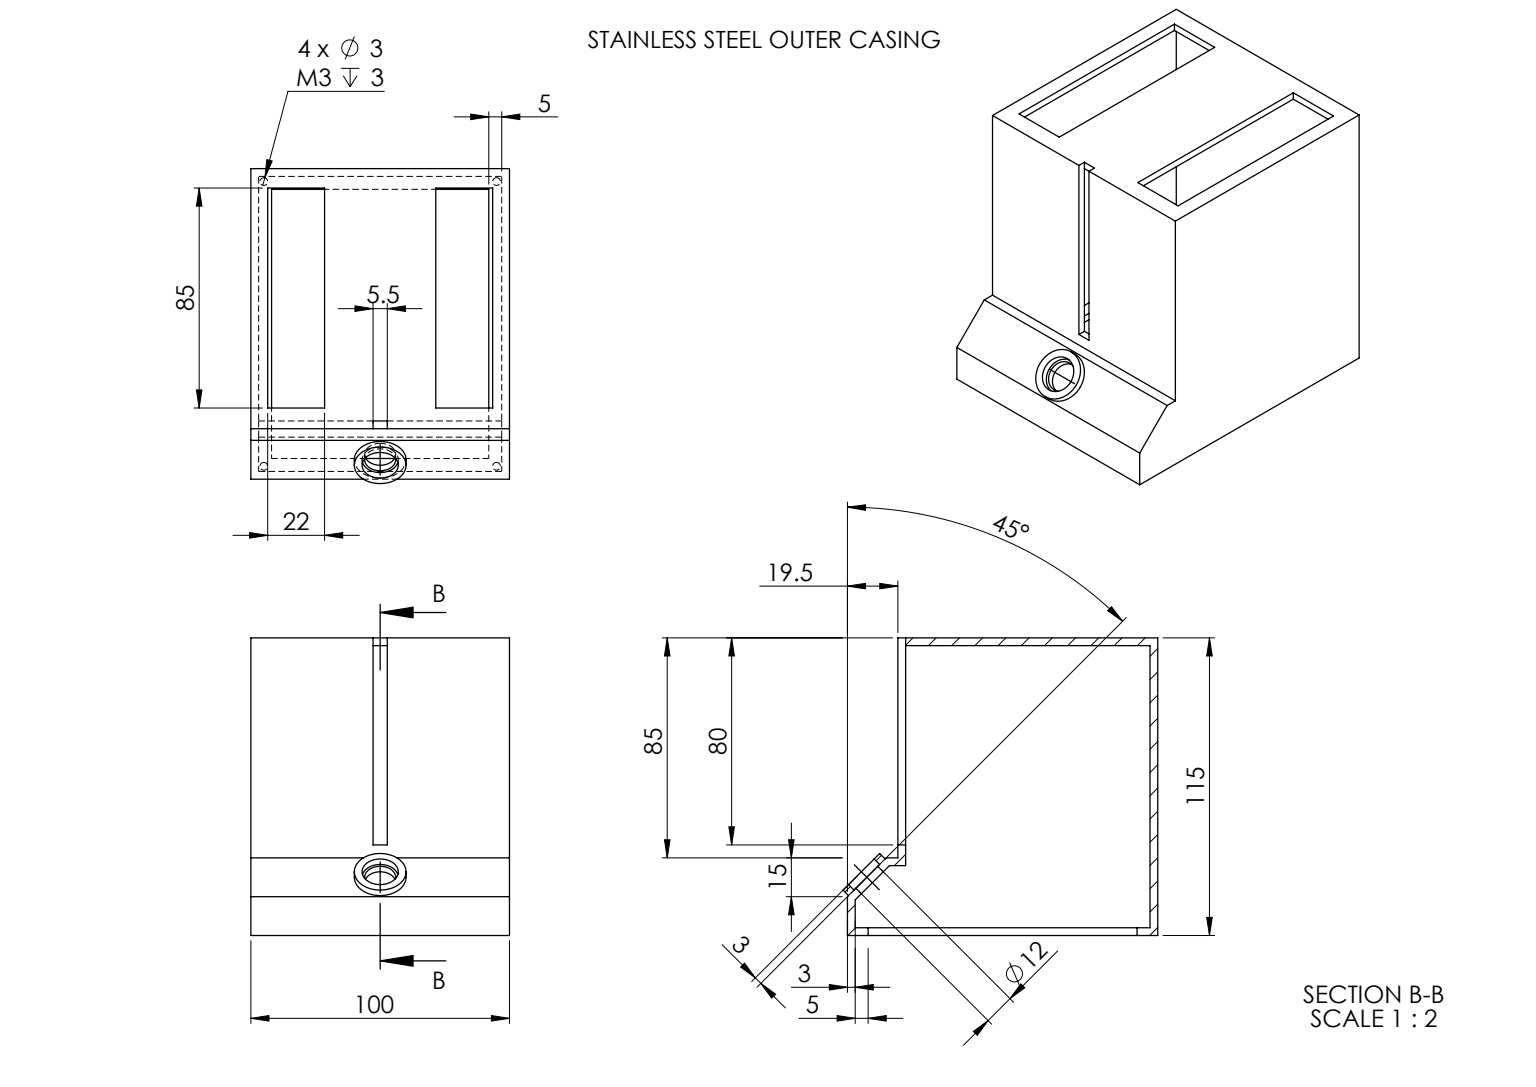
ISO-10303-21;
HEADER;
FILE_DESCRIPTION (('STEP AP214'),
    '1' );
FILE_NAME ('Stainless Steel Outer Casing.step',
    '2026-10-08T14:41:38',
    ( '' ),
    ( '' ),
    'SwSTEP 2.0',
    'SolidWorks 2026',
    '' );
FILE_SCHEMA (( 'AUTOMOTIVE_DESIGN' ));
ENDSEC;

DATA;
#7=VECTOR ( 'NONE', #15495, 1000.000000000000000 ) ;
#21=EDGE_CURVE ( 'NONE', #10175, #2143, #13600, .T. ) ;
#32=VECTOR ( 'NONE', #13036, 1000.000000000000114 ) ;
#63=VECTOR ( 'NONE', #9225, 1000.000000000000114 ) ;
#94=FACE_OUTER_BOUND ( 'NONE', #15883, .T. ) ;
#99=CARTESIAN_POINT ( 'NONE',  ( 44.99999999999997158, 6.000000000000000000, 55.00000000000000000 ) ) ;
#102=ADVANCED_FACE ( 'NONE', ( #6068 ), #4601, .T. ) ;
#110=CYLINDRICAL_SURFACE ( 'NONE', #17224, 7.000000000000001776 ) ;
#112=DIRECTION ( 'NONE',  ( 0.000000000000000000, -0.000000000000000000, 1.000000000000000000 ) ) ;
#122=ORIENTED_EDGE ( 'NONE', *, *, #7448, .F. ) ;
#133=CARTESIAN_POINT ( 'NONE',  ( -45.00000000000000000, 6.000000000000000000, 54.99999999999998579 ) ) ;
#148=EDGE_CURVE ( 'NONE', #1741, #16697, #12522, .T. ) ;
#152=CYLINDRICAL_SURFACE ( 'NONE', #8291, 1.500000000000001332 ) ;
#155=FACE_BOUND ( 'NONE', #7820, .T. ) ;
#160=VECTOR ( 'NONE', #17759, 1000.000000000000000 ) ;
#164=EDGE_CURVE ( 'NONE', #17715, #9777, #4992, .T. ) ;
#167=EDGE_LOOP ( 'NONE', ( #6125, #3258, #15700, #3937 ) ) ;
#168=ORIENTED_EDGE ( 'NONE', *, *, #9841, .T. ) ;
#174=EDGE_LOOP ( 'NONE', ( #3560, #14789, #10322, #7746, #12837, #13051 ) ) ;
#178=AXIS2_PLACEMENT_3D ( 'NONE', #10166, #16166, #2735 ) ;
#183=DIRECTION ( 'NONE',  ( 0.000000000000000000, 1.000000000000000000, 1.632680918566406793E-16 ) ) ;
#196=EDGE_LOOP ( 'NONE', ( #2060, #11072, #774, #8129 ) ) ;
#200=ORIENTED_EDGE ( 'NONE', *, *, #5789, .F. ) ;
#205=ORIENTED_EDGE ( 'NONE', *, *, #8210, .F. ) ;
#214=PLANE ( 'NONE',  #4233 ) ;
#233=LINE ( 'NONE', #4758, #9368 ) ;
#247=DIRECTION ( 'NONE',  ( 0.000000000000000000, 0.000000000000000000, 1.000000000000000000 ) ) ;
#265=ORIENTED_EDGE ( 'NONE', *, *, #5234, .T. ) ;
#269=FACE_OUTER_BOUND ( 'NONE', #16546, .T. ) ;
#283=AXIS2_PLACEMENT_3D ( 'NONE', #6653, #2040, #17044 ) ;
#289=VECTOR ( 'NONE', #11116, 1000.000000000000000 ) ;
#300=SURFACE_STYLE_USAGE ( .BOTH. , #13722 ) ;
#322=VECTOR ( 'NONE', #8447, 1000.000000000000000 ) ;
#339=DIRECTION ( 'NONE',  ( 0.000000000000000000, -1.000000000000000000, -0.000000000000000000 ) ) ;
#351=DIRECTION ( 'NONE',  ( 0.000000000000000000, 0.000000000000000000, 1.000000000000000000 ) ) ;
#403=( LENGTH_UNIT ( ) NAMED_UNIT ( * ) SI_UNIT ( .MILLI., .METRE. ) );
#413=CARTESIAN_POINT ( 'NONE',  ( 43.50000000000001421, 118.0000000000000142, 32.49999999999998579 ) ) ;
#425=CARTESIAN_POINT ( 'NONE',  ( -43.50000000000000000, 115.0000000000000000, 32.50000000000000000 ) ) ;
#431=LINE ( 'NONE', #5236, #10029 ) ;
#448=CARTESIAN_POINT ( 'NONE',  ( -41.99999999999997868, 6.000000000000005329, 51.99999999999997868 ) ) ;
#451=DIRECTION ( 'NONE',  ( 1.000000000000000000, 0.000000000000000000, 0.000000000000000000 ) ) ;
#458=EDGE_LOOP ( 'NONE', ( #8935, #13551, #15098, #14265 ) ) ;
#476=EDGE_CURVE ( 'NONE', #18462, #4631, #2600, .T. ) ;
#482=ORIENTED_EDGE ( 'NONE', *, *, #8871, .F. ) ;
#495=CARTESIAN_POINT ( 'NONE',  ( -50.00000000000001421, 17.99999999999993250, 59.99999999999997868 ) ) ;
#500=EDGE_CURVE ( 'NONE', #10686, #11531, #674, .T. ) ;
#551=LINE ( 'NONE', #3304, #5191 ) ;
#584=DIRECTION ( 'NONE',  ( -0.000000000000000000, 0.000000000000000000, -1.000000000000000000 ) ) ;
#587=VERTEX_POINT ( 'NONE', #5745 ) ;
#604=CARTESIAN_POINT ( 'NONE',  ( -50.00000000000002132, 3.000000000000000000, -60.00000000000002132 ) ) ;
#607=AXIS2_PLACEMENT_3D ( 'NONE', #1336, #7408, #13378 ) ;
#620=EDGE_CURVE ( 'NONE', #15312, #12747, #7305, .T. ) ;
#644=CARTESIAN_POINT ( 'NONE',  ( 46.99999999999998579, 16.75735931288065572, 56.99999999999997158 ) ) ;
#653=( LENGTH_UNIT ( ) NAMED_UNIT ( * ) SI_UNIT ( .MILLI., .METRE. ) );
#655=LINE ( 'NONE', #6643, #5310 ) ;
#661=VECTOR ( 'NONE', #3719, 1000.000000000000000 ) ;
#665=EDGE_CURVE ( 'NONE', #4048, #8707, #8409, .T. ) ;
#672=DIRECTION ( 'NONE',  ( -0.000000000000000000, -0.7071067811865456854, -0.7071067811865493491 ) ) ;
#674=CIRCLE ( 'NONE', #11604, 7.000000000000001776 ) ;
#675=DIRECTION ( 'NONE',  ( -1.000000000000000000, 0.000000000000000000, -2.081668171172167774E-16 ) ) ;
#709=LINE ( 'NONE', #13739, #8347 ) ;
#743=ORIENTED_EDGE ( 'NONE', *, *, #13910, .T. ) ;
#744=EDGE_CURVE ( 'NONE', #4631, #8350, #8098, .T. ) ;
#757=EDGE_CURVE ( 'NONE', #10804, #4598, #9265, .T. ) ;
#774=ORIENTED_EDGE ( 'NONE', *, *, #620, .F. ) ;
#780=CARTESIAN_POINT ( 'NONE',  ( -43.50000000000000000, 2.999000000000001442, 32.50000000000000000 ) ) ;
#791=PLANE ( 'NONE',  #8315 ) ;
#796=ORIENTED_EDGE ( 'NONE', *, *, #8690, .T. ) ;
#801=ORIENTED_EDGE ( 'NONE', *, *, #13567, .F. ) ;
#805=EDGE_CURVE ( 'NONE', #14571, #4512, #3295, .T. ) ;
#813=VECTOR ( 'NONE', #8589, 1000.000000000000000 ) ;
#814=CARTESIAN_POINT ( 'NONE',  ( -45.00000000000000000, 6.000000000000000000, 56.49999999999998579 ) ) ;
#831=LINE ( 'NONE', #11312, #7741 ) ;
#854=EDGE_LOOP ( 'NONE', ( #12884, #7574 ) ) ;
#862=LINE ( 'NONE', #12814, #6940 ) ;
#869=VERTEX_POINT ( 'NONE', #11305 ) ;
#871=ORIENTED_EDGE ( 'NONE', *, *, #3155, .F. ) ;
#884=PLANE ( 'NONE',  #9599 ) ;
#888=EDGE_CURVE ( 'NONE', #7059, #18716, #5252, .T. ) ;
#896=CARTESIAN_POINT ( 'NONE',  ( -47.00000000000001421, 118.0000000000000142, 56.99999999999997158 ) ) ;
#898=CARTESIAN_POINT ( 'NONE',  ( -21.50000000000000000, 115.0000000000000000, -52.50000000000000711 ) ) ;
#899=CARTESIAN_POINT ( 'NONE',  ( 41.99999999999997868, 3.000000000000000000, 51.99999999999997868 ) ) ;
#909=CIRCLE ( 'NONE', #3424, 1.500000000000001332 ) ;
#923=VECTOR ( 'NONE', #18178, 1000.000000000000000 ) ;
#930=SHAPE_REPRESENTATION_RELATIONSHIP ( 'NONE' , 'NONE' ,  #3576, #11772 ) ;
#948=PLANE ( 'NONE',  #3329 ) ;
#963=DIRECTION ( 'NONE',  ( 0.000000000000000000, 0.000000000000000000, -1.000000000000000000 ) ) ;
#970=DIRECTION ( 'NONE',  ( -0.000000000000000000, -1.000000000000000000, -0.000000000000000000 ) ) ;
#971=ORIENTED_EDGE ( 'NONE', *, *, #164, .F. ) ;
#972=CARTESIAN_POINT ( 'NONE',  ( -47.00000000000001421, 118.0000000000000000, 37.49999999999998579 ) ) ;
#1019=LINE ( 'NONE', #10212, #11710 ) ;
#1026=FACE_OUTER_BOUND ( 'NONE', #3398, .T. ) ;
#1031=( NAMED_UNIT ( * ) PLANE_ANGLE_UNIT ( ) SI_UNIT ( $, .RADIAN. ) );
#1041=DIRECTION ( 'NONE',  ( 0.000000000000000000, 0.000000000000000000, -1.000000000000000000 ) ) ;
#1045=ORIENTED_EDGE ( 'NONE', *, *, #6088, .F. ) ;
#1070=DIRECTION ( 'NONE',  ( 0.000000000000000000, 0.7071067811865456854, 0.7071067811865494601 ) ) ;
#1073=ORIENTED_EDGE ( 'NONE', *, *, #11613, .T. ) ;
#1109=EDGE_CURVE ( 'NONE', #7321, #12653, #14055, .T. ) ;
#1121=PLANE ( 'NONE',  #13972 ) ;
#1144=EDGE_LOOP ( 'NONE', ( #5694, #7541, #10250, #5866, #13029, #5265, #13684, #11324 ) ) ;
#1153=CARTESIAN_POINT ( 'NONE',  ( 21.50000000000001421, 115.0000000000000000, 32.49999999999998579 ) ) ;
#1162=CARTESIAN_POINT ( 'NONE',  ( -43.50000000000000711, 115.0000000000000000, -52.50000000000000711 ) ) ;
#1172=DIRECTION ( 'NONE',  ( 5.782411586589357392E-17, -0.000000000000000000, 1.000000000000000000 ) ) ;
#1188=FACE_OUTER_BOUND ( 'NONE', #1680, .T. ) ;
#1203=EDGE_CURVE ( 'NONE', #1873, #18422, #909, .T. ) ;
#1217=ADVANCED_FACE ( 'NONE', ( #5019 ), #1978, .T. ) ;
#1237=EDGE_CURVE ( 'NONE', #17810, #6948, #2262, .T. ) ;
#1244=AXIS2_PLACEMENT_3D ( 'NONE', #13571, #351, #11909 ) ;
#1254=DIRECTION ( 'NONE',  ( 3.826732013112563602E-16, -1.000000000000000000, 0.000000000000000000 ) ) ;
#1257=ORIENTED_EDGE ( 'NONE', *, *, #3159, .F. ) ;
#1287=VECTOR ( 'NONE', #5413, 1000.000000000000000 ) ;
#1300=CYLINDRICAL_SURFACE ( 'NONE', #11120, 6.000000000000000888 ) ;
#1336=CARTESIAN_POINT ( 'NONE',  ( -45.00000000000000000, 3.000000000000000000, 54.99999999999998579 ) ) ;
#1371=ORIENTED_EDGE ( 'NONE', *, *, #6399, .T. ) ;
#1405=AXIS2_PLACEMENT_3D ( 'NONE', #8749, #5726, #9920 ) ;
#1436=CARTESIAN_POINT ( 'NONE',  ( 2.749999999999979128, 118.0000000000000142, -42.68883962248118991 ) ) ;
#1440=ORIENTED_EDGE ( 'NONE', *, *, #17739, .F. ) ;
#1441=EDGE_LOOP ( 'NONE', ( #5687, #8862, #2256, #4138 ) ) ;
#1459=CARTESIAN_POINT ( 'NONE',  ( -50.00000000000001421, 118.0000000000000142, 59.99999999999997868 ) ) ;
#1461=ORIENTED_EDGE ( 'NONE', *, *, #6526, .T. ) ;
#1462=DIRECTION ( 'NONE',  ( 0.000000000000000000, 0.7071067811865494601, -0.7071067811865455743 ) ) ;
#1481=DIRECTION ( 'NONE',  ( -0.000000000000000000, -1.000000000000000000, -0.000000000000000000 ) ) ;
#1489=ADVANCED_FACE ( 'NONE', ( #19013 ), #19107, .F. ) ;
#1490=CARTESIAN_POINT ( 'NONE',  ( 21.49999999999997513, 2.999000000000001442, -52.50000000000002132 ) ) ;
#1512=LINE ( 'NONE', #15234, #5785 ) ;
#1551=DIRECTION ( 'NONE',  ( 0.000000000000000000, 0.000000000000000000, -1.000000000000000000 ) ) ;
#1590=AXIS2_PLACEMENT_3D ( 'NONE', #3065, #4546, #10504 ) ;
#1591=SHAPE_DEFINITION_REPRESENTATION ( #14745, #3576 ) ;
#1595=DIRECTION ( 'NONE',  ( 5.782411586589357392E-17, 0.000000000000000000, 1.000000000000000000 ) ) ;
#1598=CIRCLE ( 'NONE', #8768, 6.000000000000003553 ) ;
#1641=DIRECTION ( 'NONE',  ( -0.000000000000000000, -0.000000000000000000, 1.000000000000000000 ) ) ;
#1650=ORIENTED_EDGE ( 'NONE', *, *, #21, .T. ) ;
#1668=ORIENTED_EDGE ( 'NONE', *, *, #14320, .T. ) ;
#1679=DIRECTION ( 'NONE',  ( 1.000000000000000000, -0.000000000000000000, -0.000000000000000000 ) ) ;
#1680=EDGE_LOOP ( 'NONE', ( #9571, #15611, #5276, #16568 ) ) ;
#1683=FACE_BOUND ( 'NONE', #8959, .T. ) ;
#1684=FACE_OUTER_BOUND ( 'NONE', #7126, .T. ) ;
#1689=DIRECTION ( 'NONE',  ( 0.000000000000000000, 0.7071067811865456854, 0.7071067811865494601 ) ) ;
#1703=DIRECTION ( 'NONE',  ( 0.000000000000000000, 0.000000000000000000, -1.000000000000000000 ) ) ;
#1710=VERTEX_POINT ( 'NONE', #6172 ) ;
#1722=DIRECTION ( 'NONE',  ( 1.000000000000000000, 0.000000000000000000, 2.081668171172167774E-16 ) ) ;
#1730=AXIS2_PLACEMENT_3D ( 'NONE', #1783, #3543, #6587 ) ;
#1741=VERTEX_POINT ( 'NONE', #18031 ) ;
#1779=DIRECTION ( 'NONE',  ( -1.000000000000000000, 0.000000000000000000, 0.000000000000000000 ) ) ;
#1782=FACE_BOUND ( 'NONE', #2548, .T. ) ;
#1783=CARTESIAN_POINT ( 'NONE',  ( -43.50000000000000711, 2.999000000000001442, -52.50000000000000711 ) ) ;
#1791=AXIS2_PLACEMENT_3D ( 'NONE', #13713, #4815, #7646 ) ;
#1794=UNCERTAINTY_MEASURE_WITH_UNIT (LENGTH_MEASURE( 1.000000000000000082E-05 ), #15170, 'distance_accuracy_value', 'NONE');
#1852=CARTESIAN_POINT ( 'NONE',  ( -1.040834085586084257E-14, 27.62132034355962773, 54.62132034355965260 ) ) ;
#1872=PRESENTATION_STYLE_ASSIGNMENT (( #300 ) ) ;
#1873=VERTEX_POINT ( 'NONE', #16954 ) ;
#1888=CIRCLE ( 'NONE', #9998, 7.000000000000001776 ) ;
#1892=DIRECTION ( 'NONE',  ( 1.000000000000000000, 0.000000000000000000, 0.000000000000000000 ) ) ;
#1904=PLANE ( 'NONE',  #3742 ) ;
#1941=CARTESIAN_POINT ( 'NONE',  ( -41.99999999999997868, 139.6861997365471950, -52.00000000000000000 ) ) ;
#1949=CARTESIAN_POINT ( 'NONE',  ( -47.00000000000001421, 30.00000000000000355, 43.75735931288070191 ) ) ;
#1954=CARTESIAN_POINT ( 'NONE',  ( 50.00000000000000000, 3.000000000000000000, -60.00000000000000000 ) ) ;
#1956=ORIENTED_EDGE ( 'NONE', *, *, #12876, .F. ) ;
#1974=ORIENTED_EDGE ( 'NONE', *, *, #12424, .T. ) ;
#1978=PLANE ( 'NONE',  #14364 ) ;
#1979=DIRECTION ( 'NONE',  ( 0.000000000000000000, 0.000000000000000000, -1.000000000000000000 ) ) ;
#1982=CARTESIAN_POINT ( 'NONE',  ( -45.00000000000000000, 3.000000000000000000, 56.49999999999998579 ) ) ;
#1983=DIRECTION ( 'NONE',  ( 1.000000000000000000, -0.000000000000000000, -0.000000000000000000 ) ) ;
#1990=ADVANCED_FACE ( 'NONE', ( #4281 ), #10241, .F. ) ;
#1997=DIRECTION ( 'NONE',  ( 0.000000000000000000, 0.7071067811865492381, -0.7071067811865457964 ) ) ;
#1998=LINE ( 'NONE', #13856, #2231 ) ;
#2001=DIRECTION ( 'NONE',  ( -0.000000000000000000, 1.000000000000000000, -0.000000000000000000 ) ) ;
#2002=PLANE ( 'NONE',  #13642 ) ;
#2040=DIRECTION ( 'NONE',  ( -2.081668171172167774E-16, 0.000000000000000000, 1.000000000000000000 ) ) ;
#2060=ORIENTED_EDGE ( 'NONE', *, *, #1237, .F. ) ;
#2071=ADVANCED_FACE ( 'NONE', ( #11707, #17502 ), #7016, .F. ) ;
#2079=DIRECTION ( 'NONE',  ( -5.782411586589357392E-17, 0.000000000000000000, -1.000000000000000000 ) ) ;
#2081=EDGE_CURVE ( 'NONE', #18230, #8527, #14279, .T. ) ;
#2092=CARTESIAN_POINT ( 'NONE',  ( -50.00000000000002132, 33.00000000000000000, 44.99999999999999289 ) ) ;
#2096=CARTESIAN_POINT ( 'NONE',  ( -9.673552776372430100E-15, 29.74264068711928743, 48.25735931288073033 ) ) ;
#2098=AXIS2_PLACEMENT_3D ( 'NONE', #6306, #15604, #1892 ) ;
#2110=DIRECTION ( 'NONE',  ( -0.000000000000000000, -1.000000000000000000, -0.000000000000000000 ) ) ;
#2128=DIRECTION ( 'NONE',  ( 0.000000000000000000, 0.000000000000000000, -1.000000000000000000 ) ) ;
#2131=CARTESIAN_POINT ( 'NONE',  ( -1.040834085586084257E-14, -42.00099999999996214, -15.00100000000031208 ) ) ;
#2137=FACE_OUTER_BOUND ( 'NONE', #3926, .T. ) ;
#2141=LINE ( 'NONE', #8128, #7061 ) ;
#2143=VERTEX_POINT ( 'NONE', #19176 ) ;
#2159=VERTEX_POINT ( 'NONE', #12797 ) ;
#2160=DIRECTION ( 'NONE',  ( 1.000000000000000000, 0.000000000000000000, 0.000000000000000000 ) ) ;
#2167=AXIS2_PLACEMENT_3D ( 'NONE', #11686, #8658, #8949 ) ;
#2178=VECTOR ( 'NONE', #16703, 1000.000000000000000 ) ;
#2187=AXIS2_PLACEMENT_3D ( 'NONE', #4846, #17003, #15134 ) ;
#2198=EDGE_CURVE ( 'NONE', #869, #11368, #7409, .T. ) ;
#2223=LINE ( 'NONE', #1941, #12063 ) ;
#2227=VERTEX_POINT ( 'NONE', #9174 ) ;
#2231=VECTOR ( 'NONE', #5321, 1000.000000000000000 ) ;
#2255=CARTESIAN_POINT ( 'NONE',  ( 41.99999999999997868, 3.000000000000000000, 2.802245615039457371E-15 ) ) ;
#2256=ORIENTED_EDGE ( 'NONE', *, *, #1237, .T. ) ;
#2258=ORIENTED_EDGE ( 'NONE', *, *, #13660, .T. ) ;
#2262=LINE ( 'NONE', #8060, #15938 ) ;
#2270=ORIENTED_EDGE ( 'NONE', *, *, #13660, .F. ) ;
#2292=EDGE_CURVE ( 'NONE', #5477, #587, #18207, .T. ) ;
#2297=EDGE_CURVE ( 'NONE', #8527, #17051, #14859, .T. ) ;
#2344=LINE ( 'NONE', #2618, #661 ) ;
#2359=VERTEX_POINT ( 'NONE', #18499 ) ;
#2367=VECTOR ( 'NONE', #1595, 1000.000000000000000 ) ;
#2374=DIRECTION ( 'NONE',  ( 1.000000000000000000, -0.000000000000000000, 0.000000000000000000 ) ) ;
#2376=CARTESIAN_POINT ( 'NONE',  ( 46.99999999999998579, 6.000000000000000000, 56.99999999999997158 ) ) ;
#2380=ORIENTED_EDGE ( 'NONE', *, *, #2198, .F. ) ;
#2391=CARTESIAN_POINT ( 'NONE',  ( -50.00000000000002132, 118.0000000000000142, 40.49999999999997868 ) ) ;
#2394=LINE ( 'NONE', #14545, #3079 ) ;
#2401=ADVANCED_FACE ( 'NONE', ( #3680 ), #15255, .T. ) ;
#2413=DIRECTION ( 'NONE',  ( 3.826732013112563602E-16, -1.000000000000000000, 0.000000000000000000 ) ) ;
#2422=ORIENTED_EDGE ( 'NONE', *, *, #6658, .F. ) ;
#2429=ORIENTED_EDGE ( 'NONE', *, *, #6641, .T. ) ;
#2434=DIRECTION ( 'NONE',  ( -0.000000000000000000, 1.000000000000000000, -0.000000000000000000 ) ) ;
#2467=VECTOR ( 'NONE', #5678, 1000.000000000000000 ) ;
#2487=AXIS2_PLACEMENT_3D ( 'NONE', #14795, #6951, #17439 ) ;
#2507=DIRECTION ( 'NONE',  ( -8.177564888977974449E-17, -0.7071067811865495711, 0.7071067811865455743 ) ) ;
#2516=EDGE_CURVE ( 'NONE', #16874, #10684, #2394, .T. ) ;
#2519=COLOUR_RGB ( '', 0.40784314, 0.44705882, 0.49803922) ;
#2526=LINE ( 'NONE', #8412, #7509 ) ;
#2532=CARTESIAN_POINT ( 'NONE',  ( -47.00000000000001421, 30.87867965644036516, 42.87867965644034030 ) ) ;
#2538=DIRECTION ( 'NONE',  ( 0.000000000000000000, 0.000000000000000000, -1.000000000000000000 ) ) ;
#2548=EDGE_LOOP ( 'NONE', ( #7155, #3668 ) ) ;
#2552=CARTESIAN_POINT ( 'NONE',  ( 43.50000000000001421, 115.0000000000000000, 32.49999999999998579 ) ) ;
#2558=CARTESIAN_POINT ( 'NONE',  ( -41.99999999999997868, 6.000000000000005329, -52.00000000000000000 ) ) ;
#2585=DIRECTION ( 'NONE',  ( -0.000000000000000000, -1.000000000000000000, -0.000000000000000000 ) ) ;
#2586=ADVANCED_FACE ( 'NONE', ( #1026 ), #15741, .F. ) ;
#2600=LINE ( 'NONE', #12704, #11302 ) ;
#2602=CARTESIAN_POINT ( 'NONE',  ( -50.00000000000002132, 33.00000000000000000, 44.99999999999999289 ) ) ;
#2614=FACE_OUTER_BOUND ( 'NONE', #16515, .T. ) ;
#2616=CARTESIAN_POINT ( 'NONE',  ( 49.99999999999997868, 32.99999999999999289, 45.00000000000000000 ) ) ;
#2618=CARTESIAN_POINT ( 'NONE',  ( 0.000000000000000000, 3.000000000000000000, -52.00000000000000000 ) ) ;
#2623=DIRECTION ( 'NONE',  ( 9.440833060721746417E-33, 1.000000000000000000, 1.632680918566406793E-16 ) ) ;
#2629=DIRECTION ( 'NONE',  ( -8.163404592832032733E-17, 0.000000000000000000, -1.000000000000000000 ) ) ;
#2670=VERTEX_POINT ( 'NONE', #9248 ) ;
#2678=EDGE_CURVE ( 'NONE', #11126, #18238, #17229, .T. ) ;
#2681=DIRECTION ( 'NONE',  ( 0.000000000000000000, 0.000000000000000000, -1.000000000000000000 ) ) ;
#2704=CARTESIAN_POINT ( 'NONE',  ( 2.750000000000009770, 38.00000000000000000, 40.49999999999995737 ) ) ;
#2716=ORIENTED_EDGE ( 'NONE', *, *, #164, .T. ) ;
#2717=ORIENTED_EDGE ( 'NONE', *, *, #8293, .T. ) ;
#2720=DIRECTION ( 'NONE',  ( -0.000000000000000000, -1.000000000000000000, -0.000000000000000000 ) ) ;
#2729=CARTESIAN_POINT ( 'NONE',  ( -9.551088096457694952E-15, 22.67157287525377996, 59.57106781186547551 ) ) ;
#2735=DIRECTION ( 'NONE',  ( 0.000000000000000000, 0.000000000000000000, -1.000000000000000000 ) ) ;
#2744=LINE ( 'NONE', #11847, #15946 ) ;
#2747=LINE ( 'NONE', #16276, #10025 ) ;
#2749=DIRECTION ( 'NONE',  ( 0.000000000000000000, 0.7071067811865492381, -0.7071067811865457964 ) ) ;
#2751=DIRECTION ( 'NONE',  ( 0.000000000000000000, 0.000000000000000000, 1.000000000000000000 ) ) ;
#2760=ORIENTED_EDGE ( 'NONE', *, *, #18994, .F. ) ;
#2778=AXIS2_PLACEMENT_3D ( 'NONE', #6950, #9698, #15784 ) ;
#2804=AXIS2_PLACEMENT_3D ( 'NONE', #7067, #5319, #17280 ) ;
#2817=CARTESIAN_POINT ( 'NONE',  ( 44.99999999999997158, 3.000000000000000000, 55.00000000000000000 ) ) ;
#2821=PLANE ( 'NONE',  #15385 ) ;
#2842=CARTESIAN_POINT ( 'NONE',  ( 46.99999999999997868, 118.0000000000000142, 37.49999999999997868 ) ) ;
#2865=VECTOR ( 'NONE', #1641, 1000.000000000000000 ) ;
#2884=VECTOR ( 'NONE', #10918, 1000.000000000000000 ) ;
#2890=AXIS2_PLACEMENT_3D ( 'NONE', #12031, #18028, #10559 ) ;
#2899=DIRECTION ( 'NONE',  ( -0.000000000000000000, 0.7071067811865456854, 0.7071067811865493491 ) ) ;
#2901=DIRECTION ( 'NONE',  ( -0.000000000000000000, -1.000000000000000000, -0.000000000000000000 ) ) ;
#2917=DIRECTION ( 'NONE',  ( -0.000000000000000000, -1.000000000000000000, -0.000000000000000000 ) ) ;
#2933=VERTEX_POINT ( 'NONE', #3431 ) ;
#2964=EDGE_LOOP ( 'NONE', ( #14334, #15183, #19116, #15483 ) ) ;
#2965=CIRCLE ( 'NONE', #7668, 1.500000000000001332 ) ;
#2990=DIRECTION ( 'NONE',  ( 8.163404592832032733E-17, -0.000000000000000000, 1.000000000000000000 ) ) ;
#3028=CARTESIAN_POINT ( 'NONE',  ( -43.50000000000000000, 115.0000000000000000, 32.50000000000000000 ) ) ;
#3038=ADVANCED_FACE ( 'NONE', ( #18250 ), #12543, .F. ) ;
#3040=DIRECTION ( 'NONE',  ( 0.000000000000000000, -0.7071067811865455743, -0.7071067811865495711 ) ) ;
#3047=FACE_OUTER_BOUND ( 'NONE', #13827, .T. ) ;
#3057=CARTESIAN_POINT ( 'NONE',  ( -43.50000000000000711, 115.0000000000000000, -52.50000000000000711 ) ) ;
#3059=EDGE_CURVE ( 'NONE', #7257, #17715, #2526, .T. ) ;
#3065=CARTESIAN_POINT ( 'NONE',  ( 44.99999999999998579, 6.000000000000000000, -54.99999999999998579 ) ) ;
#3068=ORIENTED_EDGE ( 'NONE', *, *, #11028, .F. ) ;
#3069=CARTESIAN_POINT ( 'NONE',  ( 50.00000000000000000, 118.0000000000000142, -60.00000000000000000 ) ) ;
#3077=ADVANCED_FACE ( 'NONE', ( #5388 ), #19099, .F. ) ;
#3079=VECTOR ( 'NONE', #8379, 1000.000000000000000 ) ;
#3122=VECTOR ( 'NONE', #8349, 1000.000000000000000 ) ;
#3124=DIRECTION ( 'NONE',  ( 0.000000000000000000, -0.7071067811865455743, -0.7071067811865495711 ) ) ;
#3143=DIRECTION ( 'NONE',  ( -1.000000000000000000, 0.000000000000000000, -2.081668171172167774E-16 ) ) ;
#3145=DIRECTION ( 'NONE',  ( -0.000000000000000000, -1.000000000000000000, -0.000000000000000000 ) ) ;
#3146=ORIENTED_EDGE ( 'NONE', *, *, #9778, .T. ) ;
#3155=EDGE_CURVE ( 'NONE', #19093, #13301, #11437, .T. ) ;
#3156=LINE ( 'NONE', #4239, #13581 ) ;
#3159=EDGE_CURVE ( 'NONE', #11531, #10686, #1888, .T. ) ;
#3164=VECTOR ( 'NONE', #15871, 1000.000000000000000 ) ;
#3182=VECTOR ( 'NONE', #6048, 1000.000000000000000 ) ;
#3207=VERTEX_POINT ( 'NONE', #16153 ) ;
#3221=ORIENTED_EDGE ( 'NONE', *, *, #2297, .F. ) ;
#3224=EDGE_LOOP ( 'NONE', ( #1461, #3421, #10604, #3377, #7859, #9045, #1956 ) ) ;
#3243=CARTESIAN_POINT ( 'NONE',  ( 44.99999999999998579, 3.000000000000000000, -53.49999999999998579 ) ) ;
#3244=ORIENTED_EDGE ( 'NONE', *, *, #12564, .F. ) ;
#3246=ORIENTED_EDGE ( 'NONE', *, *, #11267, .F. ) ;
#3247=CARTESIAN_POINT ( 'NONE',  ( -21.50000000000000000, 2.999000000000001442, 32.50000000000000000 ) ) ;
#3249=DIRECTION ( 'NONE',  ( -0.000000000000000000, -1.000000000000000000, -0.000000000000000000 ) ) ;
#3258=ORIENTED_EDGE ( 'NONE', *, *, #12894, .T. ) ;
#3262=ORIENTED_EDGE ( 'NONE', *, *, #888, .F. ) ;
#3271=ORIENTED_EDGE ( 'NONE', *, *, #13416, .F. ) ;
#3292=ADVANCED_FACE ( 'NONE', ( #4250 ), #17581, .F. ) ;
#3295=LINE ( 'NONE', #448, #8119 ) ;
#3304=CARTESIAN_POINT ( 'NONE',  ( -50.00000000000002132, 115.0000000000000000, 37.49999999999997868 ) ) ;
#3320=EDGE_LOOP ( 'NONE', ( #3991, #6363, #14479, #13024 ) ) ;
#3329=AXIS2_PLACEMENT_3D ( 'NONE', #3804, #5460, #14100 ) ;
#3352=FACE_BOUND ( 'NONE', #3535, .T. ) ;
#3364=ORIENTED_EDGE ( 'NONE', *, *, #6641, .F. ) ;
#3377=ORIENTED_EDGE ( 'NONE', *, *, #19080, .T. ) ;
#3388=FACE_BOUND ( 'NONE', #10760, .T. ) ;
#3398=EDGE_LOOP ( 'NONE', ( #9677, #5414, #14418, #16563 ) ) ;
#3421=ORIENTED_EDGE ( 'NONE', *, *, #9621, .F. ) ;
#3424=AXIS2_PLACEMENT_3D ( 'NONE', #11166, #3542, #6681 ) ;
#3431=CARTESIAN_POINT ( 'NONE',  ( -44.99999999999998579, 3.000000000000000000, -53.50000000000000000 ) ) ;
#3432=ORIENTED_EDGE ( 'NONE', *, *, #7464, .F. ) ;
#3443=PLANE ( 'NONE',  #1730 ) ;
#3450=DIRECTION ( 'NONE',  ( 1.000000000000000000, 0.000000000000000000, 0.000000000000000000 ) ) ;
#3454=PLANE ( 'NONE',  #2098 ) ;
#3466=CARTESIAN_POINT ( 'NONE',  ( 0.000000000000000000, 115.0000000000000000, 0.000000000000000000 ) ) ;
#3495=EDGE_CURVE ( 'NONE', #4095, #2670, #5335, .T. ) ;
#3500=ORIENTED_EDGE ( 'NONE', *, *, #16011, .F. ) ;
#3527=ORIENTED_EDGE ( 'NONE', *, *, #10674, .T. ) ;
#3532=CARTESIAN_POINT ( 'NONE',  ( 43.49999999999997868, 2.999000000000001442, -52.50000000000002132 ) ) ;
#3535=EDGE_LOOP ( 'NONE', ( #10998, #6507, #12058, #6157 ) ) ;
#3540=LINE ( 'NONE', #6486, #16321 ) ;
#3542=DIRECTION ( 'NONE',  ( -0.000000000000000000, -1.000000000000000000, -0.000000000000000000 ) ) ;
#3543=DIRECTION ( 'NONE',  ( 0.000000000000000000, 0.000000000000000000, -1.000000000000000000 ) ) ;
#3560=ORIENTED_EDGE ( 'NONE', *, *, #19080, .F. ) ;
#3576=SHAPE_REPRESENTATION ( 'Stainless Steel Outer Casing', ( #1791 ), #15487 ) ;
#3590=VERTEX_POINT ( 'NONE', #7779 ) ;
#3594=LINE ( 'NONE', #14182, #8318 ) ;
#3618=AXIS2_PLACEMENT_3D ( 'NONE', #11931, #17924, #2128 ) ;
#3628=EDGE_CURVE ( 'NONE', #15935, #12535, #7883, .T. ) ;
#3633=CARTESIAN_POINT ( 'NONE',  ( -50.00000000000002132, 16.75735931288065572, 56.99999999999997158 ) ) ;
#3661=VECTOR ( 'NONE', #1983, 1000.000000000000000 ) ;
#3663=PLANE ( 'NONE',  #8574 ) ;
#3668=ORIENTED_EDGE ( 'NONE', *, *, #13567, .T. ) ;
#3680=FACE_OUTER_BOUND ( 'NONE', #8622, .T. ) ;
#3691=DIRECTION ( 'NONE',  ( 4.081702296416016490E-16, -0.000000000000000000, 1.000000000000000000 ) ) ;
#3694=ORIENTED_EDGE ( 'NONE', *, *, #14060, .F. ) ;
#3713=AXIS2_PLACEMENT_3D ( 'NONE', #18895, #17322, #1041 ) ;
#3719=DIRECTION ( 'NONE',  ( 1.000000000000000000, -0.000000000000000000, 0.000000000000000000 ) ) ;
#3732=FACE_OUTER_BOUND ( 'NONE', #12990, .T. ) ;
#3742=AXIS2_PLACEMENT_3D ( 'NONE', #3466, #5040, #15432 ) ;
#3769=CARTESIAN_POINT ( 'NONE',  ( 44.99999999999997158, 3.000000000000000000, 56.50000000000000000 ) ) ;
#3776=EDGE_CURVE ( 'NONE', #15097, #4424, #9989, .T. ) ;
#3787=VECTOR ( 'NONE', #14568, 1000.000000000000000 ) ;
#3788=SURFACE_SIDE_STYLE ('',( #18696 ) ) ;
#3804=CARTESIAN_POINT ( 'NONE',  ( -41.99999999999997868, 139.6861997365471950, -52.00000000000000000 ) ) ;
#3819=DIRECTION ( 'NONE',  ( -0.000000000000000000, 0.7071067811865456854, 0.7071067811865493491 ) ) ;
#3829=CIRCLE ( 'NONE', #14785, 1.500000000000001332 ) ;
#3846=EDGE_CURVE ( 'NONE', #6167, #8073, #2747, .T. ) ;
#3882=EDGE_CURVE ( 'NONE', #12628, #17940, #15109, .T. ) ;
#3887=CARTESIAN_POINT ( 'NONE',  ( -50.00000000000002132, 118.0000000000000142, -60.00000000000002132 ) ) ;
#3889=LINE ( 'NONE', #18797, #9428 ) ;
#3892=ORIENTED_EDGE ( 'NONE', *, *, #148, .T. ) ;
#3909=VERTEX_POINT ( 'NONE', #7355 ) ;
#3912=DIRECTION ( 'NONE',  ( -0.000000000000000000, 0.000000000000000000, 1.000000000000000000 ) ) ;
#3922=ORIENTED_EDGE ( 'NONE', *, *, #19308, .F. ) ;
#3926=EDGE_LOOP ( 'NONE', ( #19216, #17342, #11741, #12693 ) ) ;
#3931=AXIS2_PLACEMENT_3D ( 'NONE', #5217, #1070, #13018 ) ;
#3937=ORIENTED_EDGE ( 'NONE', *, *, #4967, .F. ) ;
#3939=CARTESIAN_POINT ( 'NONE',  ( -50.00000000000002132, 115.0000000000000000, 37.49999999999997868 ) ) ;
#3973=AXIS2_PLACEMENT_3D ( 'NONE', #99, #16171, #6081 ) ;
#3974=PRESENTATION_STYLE_ASSIGNMENT (( #6726 ) ) ;
#3981=CARTESIAN_POINT ( 'NONE',  ( -41.99999999999997868, 3.000000000000002665, -52.00000000000000000 ) ) ;
#3991=ORIENTED_EDGE ( 'NONE', *, *, #5773, .T. ) ;
#3999=DIRECTION ( 'NONE',  ( 0.000000000000000000, 0.000000000000000000, -1.000000000000000000 ) ) ;
#4001=DIRECTION ( 'NONE',  ( -0.000000000000000000, 1.000000000000000000, -0.000000000000000000 ) ) ;
#4026=ORIENTED_EDGE ( 'NONE', *, *, #4115, .F. ) ;
#4028=EDGE_LOOP ( 'NONE', ( #18743, #6609, #16533, #16847 ) ) ;
#4041=VERTEX_POINT ( 'NONE', #3243 ) ;
#4048=VERTEX_POINT ( 'NONE', #15207 ) ;
#4051=MANIFOLD_SOLID_BREP ( 'Extrude-Thin1', #6669 ) ;
#4071=AXIS2_PLACEMENT_3D ( 'NONE', #5795, #5997, #11854 ) ;
#4079=DIRECTION ( 'NONE',  ( 1.000000000000000000, 0.000000000000000000, 0.000000000000000000 ) ) ;
#4091=EDGE_CURVE ( 'NONE', #12028, #12628, #10065, .T. ) ;
#4095=VERTEX_POINT ( 'NONE', #9693 ) ;
#4104=EDGE_CURVE ( 'NONE', #15084, #7321, #15686, .T. ) ;
#4115=EDGE_CURVE ( 'NONE', #4598, #2143, #2344, .T. ) ;
#4130=EDGE_CURVE ( 'NONE', #2143, #7552, #14487, .T. ) ;
#4132=ORIENTED_EDGE ( 'NONE', *, *, #18875, .T. ) ;
#4138=ORIENTED_EDGE ( 'NONE', *, *, #18213, .F. ) ;
#4142=CIRCLE ( 'NONE', #16352, 1.500000000000001332 ) ;
#4152=PRODUCT_DEFINITION_CONTEXT ( 'detailed design', #12696, 'design' ) ;
#4165=PRODUCT_DEFINITION ( 'UNKNOWN', '', #15195, #4152 ) ;
#4168=CARTESIAN_POINT ( 'NONE',  ( 44.99999999999997158, 6.000000000000000000, 55.00000000000000000 ) ) ;
#4170=CARTESIAN_POINT ( 'NONE',  ( -43.50000000000000711, 118.0000000000000142, -52.50000000000000711 ) ) ;
#4184=DIRECTION ( 'NONE',  ( 0.000000000000000000, 0.000000000000000000, -1.000000000000000000 ) ) ;
#4197=PLANE ( 'NONE',  #12588 ) ;
#4202=ORIENTED_EDGE ( 'NONE', *, *, #21, .F. ) ;
#4203=VECTOR ( 'NONE', #16316, 1000.000000000000000 ) ;
#4233=AXIS2_PLACEMENT_3D ( 'NONE', #13333, #6394, #9222 ) ;
#4239=CARTESIAN_POINT ( 'NONE',  ( 2.750000000000009770, 38.00000000000000000, 37.49999999999995737 ) ) ;
#4245=VECTOR ( 'NONE', #7275, 1000.000000000000000 ) ;
#4250=FACE_OUTER_BOUND ( 'NONE', #11335, .T. ) ;
#4266=DIRECTION ( 'NONE',  ( -1.156482317317871725E-16, 0.000000000000000000, 1.000000000000000000 ) ) ;
#4267=EDGE_LOOP ( 'NONE', ( #14611, #10667, #15284, #14682 ) ) ;
#4281=FACE_OUTER_BOUND ( 'NONE', #7993, .T. ) ;
#4288=ORIENTED_EDGE ( 'NONE', *, *, #17165, .T. ) ;
#4317=ORIENTED_EDGE ( 'NONE', *, *, #18004, .T. ) ;
#4333=ADVANCED_FACE ( 'NONE', ( #10458 ), #2821, .F. ) ;
#4337=CARTESIAN_POINT ( 'NONE',  ( -21.50000000000000000, 115.0000000000000000, 32.50000000000000000 ) ) ;
#4394=EDGE_CURVE ( 'NONE', #6468, #7257, #18324, .T. ) ;
#4412=VERTEX_POINT ( 'NONE', #1949 ) ;
#4413=ORIENTED_EDGE ( 'NONE', *, *, #2516, .F. ) ;
#4416=DIRECTION ( 'NONE',  ( -1.156482317317871725E-16, 0.000000000000000000, 1.000000000000000000 ) ) ;
#4419=ORIENTED_EDGE ( 'NONE', *, *, #17019, .F. ) ;
#4424=VERTEX_POINT ( 'NONE', #12327 ) ;
#4428=AXIS2_PLACEMENT_3D ( 'NONE', #18521, #10948, #183 ) ;
#4440=DIRECTION ( 'NONE',  ( -0.000000000000000000, 0.7071067811865456854, 0.7071067811865494601 ) ) ;
#4448=ADVANCED_FACE ( 'NONE', ( #8029 ), #13797, .F. ) ;
#4453=EDGE_LOOP ( 'NONE', ( #7759, #12043, #971, #16465 ) ) ;
#4470=VECTOR ( 'NONE', #8030, 1000.000000000000000 ) ;
#4477=FACE_OUTER_BOUND ( 'NONE', #3320, .T. ) ;
#4498=DIRECTION ( 'NONE',  ( -0.000000000000000000, -0.7071067811865456854, -0.7071067811865494601 ) ) ;
#4511=LINE ( 'NONE', #3028, #6746 ) ;
#4512=VERTEX_POINT ( 'NONE', #13599 ) ;
#4527=FACE_OUTER_BOUND ( 'NONE', #15033, .T. ) ;
#4535=CARTESIAN_POINT ( 'NONE',  ( -9.183694056713489507E-15, 20.55025253169413091, 61.69238815542511389 ) ) ;
#4546=DIRECTION ( 'NONE',  ( -0.000000000000000000, -1.000000000000000000, -0.000000000000000000 ) ) ;
#4579=CARTESIAN_POINT ( 'NONE',  ( 47.00000000000000000, 6.000000000000000000, -56.99999999999999289 ) ) ;
#4598=VERTEX_POINT ( 'NONE', #3981 ) ;
#4601=PLANE ( 'NONE',  #2890 ) ;
#4629=EDGE_CURVE ( 'NONE', #11279, #6468, #11223, .T. ) ;
#4630=CARTESIAN_POINT ( 'NONE',  ( 49.99999999999998579, 118.0000000000000142, 59.99999999999997868 ) ) ;
#4631=VERTEX_POINT ( 'NONE', #5454 ) ;
#4654=CARTESIAN_POINT ( 'NONE',  ( -47.00000000000001421, 6.000000000000000000, 56.99999999999997158 ) ) ;
#4695=ORIENTED_EDGE ( 'NONE', *, *, #11029, .T. ) ;
#4731=CARTESIAN_POINT ( 'NONE',  ( -21.50000000000000000, 118.0000000000000142, -52.50000000000000711 ) ) ;
#4740=EDGE_LOOP ( 'NONE', ( #18121, #19348, #12434, #16593 ) ) ;
#4750=CARTESIAN_POINT ( 'NONE',  ( -1.040834085586084257E-14, 34.69238815542512100, 47.55025253169419841 ) ) ;
#4757=ORIENTED_EDGE ( 'NONE', *, *, #805, .T. ) ;
#4758=CARTESIAN_POINT ( 'NONE',  ( -41.99999999999997868, 139.6861997365471950, 51.99999999999997868 ) ) ;
#4766=CARTESIAN_POINT ( 'NONE',  ( 21.50000000000001421, 2.999000000000001442, 32.49999999999998579 ) ) ;
#4781=CARTESIAN_POINT ( 'NONE',  ( -44.99999999999998579, 3.000000000000000000, -55.00000000000000000 ) ) ;
#4784=AXIS2_PLACEMENT_3D ( 'NONE', #12124, #4498, #18023 ) ;
#4815=DIRECTION ( 'NONE',  ( 0.000000000000000000, 0.000000000000000000, 1.000000000000000000 ) ) ;
#4826=ORIENTED_EDGE ( 'NONE', *, *, #16711, .T. ) ;
#4844=DIRECTION ( 'NONE',  ( -0.000000000000000000, -1.000000000000000000, -0.000000000000000000 ) ) ;
#4846=CARTESIAN_POINT ( 'NONE',  ( 2.749999999999979128, 118.0000000000000142, -42.68883962248118991 ) ) ;
#4852=DIRECTION ( 'NONE',  ( 0.000000000000000000, 0.7071067811865456854, 0.7071067811865494601 ) ) ;
#4859=MECHANICAL_DESIGN_GEOMETRIC_PRESENTATION_REPRESENTATION('',(#7343),#8585);
#4894=CARTESIAN_POINT ( 'NONE',  ( 43.49999999999997868, 115.0000000000000000, -52.50000000000002132 ) ) ;
#4909=ORIENTED_EDGE ( 'NONE', *, *, #14060, .T. ) ;
#4919=FILL_AREA_STYLE ('',( #18254 ) ) ;
#4921=CIRCLE ( 'NONE', #8348, 10.00000000000000178 ) ;
#4927=DIRECTION ( 'NONE',  ( -0.000000000000000000, -1.000000000000000000, -0.000000000000000000 ) ) ;
#4936=CIRCLE ( 'NONE', #3973, 1.500000000000001332 ) ;
#4967=EDGE_CURVE ( 'NONE', #15935, #17810, #11074, .T. ) ;
#4992=LINE ( 'NONE', #16951, #4470 ) ;
#4996=CYLINDRICAL_SURFACE ( 'NONE', #9726, 10.00000000000000000 ) ;
#5000=ORIENTED_EDGE ( 'NONE', *, *, #9256, .F. ) ;
#5017=LINE ( 'NONE', #972, #14753 ) ;
#5019=FACE_OUTER_BOUND ( 'NONE', #1144, .T. ) ;
#5026=AXIS2_PLACEMENT_3D ( 'NONE', #3532, #584, #8050 ) ;
#5032=VECTOR ( 'NONE', #14942, 1000.000000000000000 ) ;
#5040=DIRECTION ( 'NONE',  ( 0.000000000000000000, 1.000000000000000000, 0.000000000000000000 ) ) ;
#5081=APPLICATION_CONTEXT ( 'automotive_design' ) ;
#5118=PLANE ( 'NONE',  #13506 ) ;
#5119=ADVANCED_FACE ( 'NONE', ( #15971, #11444 ), #13011, .T. ) ;
#5128=LINE ( 'NONE', #11081, #15557 ) ;
#5143=DIRECTION ( 'NONE',  ( 0.000000000000000000, -0.000000000000000000, 1.000000000000000000 ) ) ;
#5163=COLOUR_RGB ( '', 0.40784314, 0.44705882, 0.49803922) ;
#5164=CIRCLE ( 'NONE', #1405, 1.500000000000001332 ) ;
#5167=DIRECTION ( 'NONE',  ( -4.088782444488986608E-17, 0.7071067811865495711, -0.7071067811865455743 ) ) ;
#5188=VECTOR ( 'NONE', #13405, 1000.000000000000000 ) ;
#5191=VECTOR ( 'NONE', #9273, 1000.000000000000000 ) ;
#5208=DIRECTION ( 'NONE',  ( -1.000000000000000000, -0.000000000000000000, -0.000000000000000000 ) ) ;
#5217=CARTESIAN_POINT ( 'NONE',  ( -1.040834085586084257E-14, 25.49999999999998934, 52.50000000000000711 ) ) ;
#5233=CARTESIAN_POINT ( 'NONE',  ( 49.99999999999998579, 3.000000000000000000, 59.99999999999997868 ) ) ;
#5234=EDGE_CURVE ( 'NONE', #18711, #14054, #8609, .T. ) ;
#5236=CARTESIAN_POINT ( 'NONE',  ( 44.99999999999997158, 3.000000000000000000, 56.50000000000000000 ) ) ;
#5252=LINE ( 'NONE', #2391, #10272 ) ;
#5262=CARTESIAN_POINT ( 'NONE',  ( -45.00000000000000000, 3.000000000000000000, 53.49999999999998579 ) ) ;
#5265=ORIENTED_EDGE ( 'NONE', *, *, #11090, .F. ) ;
#5267=DIRECTION ( 'NONE',  ( -4.898042755699219393E-16, 0.000000000000000000, -1.000000000000000000 ) ) ;
#5276=ORIENTED_EDGE ( 'NONE', *, *, #5604, .T. ) ;
#5285=DIRECTION ( 'NONE',  ( -8.177564888977974449E-17, -0.7071067811865495711, 0.7071067811865455743 ) ) ;
#5291=LINE ( 'NONE', #9878, #11557 ) ;
#5310=VECTOR ( 'NONE', #5167, 1000.000000000000114 ) ;
#5315=VERTEX_POINT ( 'NONE', #13302 ) ;
#5317=CARTESIAN_POINT ( 'NONE',  ( -47.00000000000001421, 30.00000000000000355, 37.49999999999996447 ) ) ;
#5319=DIRECTION ( 'NONE',  ( 1.000000000000000000, 0.000000000000000000, -5.782411586589357392E-17 ) ) ;
#5321=DIRECTION ( 'NONE',  ( -0.000000000000000000, -1.000000000000000000, -0.000000000000000000 ) ) ;
#5325=EDGE_CURVE ( 'NONE', #4512, #10175, #5871, .T. ) ;
#5328=EDGE_CURVE ( 'NONE', #5928, #6595, #18465, .T. ) ;
#5335=CIRCLE ( 'NONE', #1590, 1.500000000000001332 ) ;
#5350=CARTESIAN_POINT ( 'NONE',  ( -44.99999999999998579, 3.000000000000000000, -56.50000000000000000 ) ) ;
#5356=VECTOR ( 'NONE', #18528, 1000.000000000000000 ) ;
#5373=CARTESIAN_POINT ( 'NONE',  ( 21.49999999999997513, 118.0000000000000142, -52.50000000000002132 ) ) ;
#5388=FACE_OUTER_BOUND ( 'NONE', #11150, .T. ) ;
#5390=CARTESIAN_POINT ( 'NONE',  ( -9.673552776372430100E-15, -37.75835931288066405, -19.24364068711958708 ) ) ;
#5413=DIRECTION ( 'NONE',  ( 1.000000000000000000, 0.000000000000000000, 0.000000000000000000 ) ) ;
#5414=ORIENTED_EDGE ( 'NONE', *, *, #1203, .F. ) ;
#5418=LINE ( 'NONE', #11374, #160 ) ;
#5445=CARTESIAN_POINT ( 'NONE',  ( -50.00000000000001421, 3.000000000000000000, 59.99999999999997868 ) ) ;
#5454=CARTESIAN_POINT ( 'NONE',  ( 47.00000000000000000, 115.0000000000000000, -56.99999999999999289 ) ) ;
#5460=DIRECTION ( 'NONE',  ( -0.000000000000000000, 0.000000000000000000, 1.000000000000000000 ) ) ;
#5477=VERTEX_POINT ( 'NONE', #13896 ) ;
#5481=ADVANCED_FACE ( 'NONE', ( #2137 ), #11047, .F. ) ;
#5488=VECTOR ( 'NONE', #2374, 1000.000000000000000 ) ;
#5525=LINE ( 'NONE', #14536, #13899 ) ;
#5529=CIRCLE ( 'NONE', #11459, 7.000000000000004441 ) ;
#5568=DIRECTION ( 'NONE',  ( 0.000000000000000000, -1.000000000000000000, 0.000000000000000000 ) ) ;
#5583=CARTESIAN_POINT ( 'NONE',  ( 21.50000000000001421, 2.999000000000001442, 32.49999999999998579 ) ) ;
#5592=LINE ( 'NONE', #17549, #14687 ) ;
#5600=CARTESIAN_POINT ( 'NONE',  ( -50.00000000000002132, 118.0000000000000142, -60.00000000000002132 ) ) ;
#5604=EDGE_CURVE ( 'NONE', #2159, #12653, #14765, .T. ) ;
#5660=ORIENTED_EDGE ( 'NONE', *, *, #11029, .F. ) ;
#5662=ORIENTED_EDGE ( 'NONE', *, *, #19308, .T. ) ;
#5675=ADVANCED_FACE ( 'NONE', ( #10434 ), #19371, .F. ) ;
#5678=DIRECTION ( 'NONE',  ( 1.000000000000000000, -0.000000000000000000, 0.000000000000000000 ) ) ;
#5686=FACE_OUTER_BOUND ( 'NONE', #15180, .T. ) ;
#5687=ORIENTED_EDGE ( 'NONE', *, *, #6658, .T. ) ;
#5694=ORIENTED_EDGE ( 'NONE', *, *, #19018, .F. ) ;
#5726=DIRECTION ( 'NONE',  ( -0.000000000000000000, -1.000000000000000000, -0.000000000000000000 ) ) ;
#5735=CARTESIAN_POINT ( 'NONE',  ( -43.50000000000000000, 118.0000000000000142, 32.50000000000000000 ) ) ;
#5745=CARTESIAN_POINT ( 'NONE',  ( 2.749999999999980460, 115.0000000000000000, 37.49999999999997158 ) ) ;
#5752=ORIENTED_EDGE ( 'NONE', *, *, #2081, .F. ) ;
#5758=VERTEX_POINT ( 'NONE', #18928 ) ;
#5773=EDGE_CURVE ( 'NONE', #13043, #11279, #15799, .T. ) ;
#5783=VERTEX_POINT ( 'NONE', #15889 ) ;
#5785=VECTOR ( 'NONE', #9246, 1000.000000000000000 ) ;
#5789=EDGE_CURVE ( 'NONE', #2227, #587, #5592, .T. ) ;
#5795=CARTESIAN_POINT ( 'NONE',  ( -50.00000000000002132, 118.0000000000000142, -60.00000000000002132 ) ) ;
#5800=AXIS2_PLACEMENT_3D ( 'NONE', #7962, #4927, #17074 ) ;
#5830=ADVANCED_FACE ( 'NONE', ( #5990, #7259 ), #12051, .F. ) ;
#5860=ORIENTED_EDGE ( 'NONE', *, *, #4091, .F. ) ;
#5866=ORIENTED_EDGE ( 'NONE', *, *, #15046, .T. ) ;
#5871=LINE ( 'NONE', #18030, #9675 ) ;
#5875=PLANE ( 'NONE',  #18021 ) ;
#5881=EDGE_CURVE ( 'NONE', #5758, #18462, #15001, .T. ) ;
#5883=ORIENTED_EDGE ( 'NONE', *, *, #620, .T. ) ;
#5893=ORIENTED_EDGE ( 'NONE', *, *, #500, .F. ) ;
#5895=ORIENTED_EDGE ( 'NONE', *, *, #10385, .F. ) ;
#5915=VERTEX_POINT ( 'NONE', #16271 ) ;
#5928=VERTEX_POINT ( 'NONE', #10577 ) ;
#5965=ORIENTED_EDGE ( 'NONE', *, *, #6399, .F. ) ;
#5977=STYLED_ITEM ( 'NONE', ( #1872 ), #4051 ) ;
#5990=FACE_BOUND ( 'NONE', #854, .T. ) ;
#5992=EDGE_CURVE ( 'NONE', #6167, #9683, #2744, .T. ) ;
#5997=DIRECTION ( 'NONE',  ( 1.000000000000000000, 0.000000000000000000, -5.782411586589357392E-17 ) ) ;
#5998=PRODUCT ( 'Stainless Steel Outer Casing', 'Stainless Steel Outer Casing', '', ( #17564 ) ) ;
#6018=AXIS2_PLACEMENT_3D ( 'NONE', #2817, #2720, #11724 ) ;
#6045=DIRECTION ( 'NONE',  ( 0.000000000000000000, 0.7071067811865456854, 0.7071067811865494601 ) ) ;
#6046=CARTESIAN_POINT ( 'NONE',  ( -1.040834085586084257E-14, -46.24364068711926024, -10.75835931288103886 ) ) ;
#6048=DIRECTION ( 'NONE',  ( -1.000000000000000000, 0.000000000000000000, 0.000000000000000000 ) ) ;
#6068=FACE_OUTER_BOUND ( 'NONE', #16474, .T. ) ;
#6081=DIRECTION ( 'NONE',  ( 0.000000000000000000, 0.000000000000000000, -1.000000000000000000 ) ) ;
#6082=ORIENTED_EDGE ( 'NONE', *, *, #8871, .T. ) ;
#6088=EDGE_CURVE ( 'NONE', #1710, #12028, #655, .T. ) ;
#6125=ORIENTED_EDGE ( 'NONE', *, *, #3628, .T. ) ;
#6138=PLANE ( 'NONE',  #7019 ) ;
#6142=DIRECTION ( 'NONE',  ( 0.000000000000000000, 1.000000000000000000, 0.000000000000000000 ) ) ;
#6152=ORIENTED_EDGE ( 'NONE', *, *, #6863, .F. ) ;
#6157=ORIENTED_EDGE ( 'NONE', *, *, #5325, .F. ) ;
#6167=VERTEX_POINT ( 'NONE', #3069 ) ;
#6172=CARTESIAN_POINT ( 'NONE',  ( -50.00000000000001421, 17.99999999999993250, 59.99999999999997868 ) ) ;
#6182=EDGE_LOOP ( 'NONE', ( #15085, #6152, #8159, #5895 ) ) ;
#6234=VECTOR ( 'NONE', #2899, 1000.000000000000114 ) ;
#6251=EDGE_LOOP ( 'NONE', ( #9186, #1440, #16360, #2422 ) ) ;
#6262=DIRECTION ( 'NONE',  ( 0.000000000000000000, -1.000000000000000000, 0.000000000000000000 ) ) ;
#6263=ORIENTED_EDGE ( 'NONE', *, *, #18213, .T. ) ;
#6272=EDGE_LOOP ( 'NONE', ( #7222, #15779, #5883, #15459 ) ) ;
#6288=( NAMED_UNIT ( * ) PLANE_ANGLE_UNIT ( ) SI_UNIT ( $, .RADIAN. ) );
#6302=CARTESIAN_POINT ( 'NONE',  ( -1.040834085586084257E-14, 25.49999999999998934, 52.50000000000000000 ) ) ;
#6306=CARTESIAN_POINT ( 'NONE',  ( -50.00000000000002132, 30.87867965644036516, 42.87867965644034030 ) ) ;
#6323=CARTESIAN_POINT ( 'NONE',  ( -50.00000000000002132, 30.00000000000000355, 59.99999999999997868 ) ) ;
#6327=ADVANCED_FACE ( 'NONE', ( #9149 ), #11002, .T. ) ;
#6352=ORIENTED_EDGE ( 'NONE', *, *, #4130, .T. ) ;
#6363=ORIENTED_EDGE ( 'NONE', *, *, #10106, .T. ) ;
#6394=DIRECTION ( 'NONE',  ( 0.000000000000000000, -1.000000000000000000, -0.000000000000000000 ) ) ;
#6399=EDGE_CURVE ( 'NONE', #14571, #10804, #233, .T. ) ;
#6419=ADVANCED_FACE ( 'NONE', ( #16801, #15324, #16898 ), #1904, .F. ) ;
#6468=VERTEX_POINT ( 'NONE', #12756 ) ;
#6478=EDGE_LOOP ( 'NONE', ( #1257, #5893 ) ) ;
#6481=( NAMED_UNIT ( * ) SI_UNIT ( $, .STERADIAN. ) SOLID_ANGLE_UNIT ( ) );
#6486=CARTESIAN_POINT ( 'NONE',  ( -2.750000000000020872, 118.0000000000000142, 37.49999999999997158 ) ) ;
#6499=EDGE_CURVE ( 'NONE', #4424, #9683, #15805, .T. ) ;
#6507=ORIENTED_EDGE ( 'NONE', *, *, #11406, .F. ) ;
#6515=DIRECTION ( 'NONE',  ( 0.000000000000000000, 0.000000000000000000, -1.000000000000000000 ) ) ;
#6523=ADVANCED_FACE ( 'NONE', ( #15998 ), #12848, .T. ) ;
#6526=EDGE_CURVE ( 'NONE', #3207, #7196, #8541, .T. ) ;
#6552=VERTEX_POINT ( 'NONE', #8173 ) ;
#6565=AXIS2_PLACEMENT_3D ( 'NONE', #17973, #11782, #8944 ) ;
#6567=ORIENTED_EDGE ( 'NONE', *, *, #18266, .T. ) ;
#6581=ORIENTED_EDGE ( 'NONE', *, *, #8836, .T. ) ;
#6587=DIRECTION ( 'NONE',  ( -1.000000000000000000, 0.000000000000000000, -0.000000000000000000 ) ) ;
#6592=LINE ( 'NONE', #413, #3661 ) ;
#6595=VERTEX_POINT ( 'NONE', #15715 ) ;
#6608=LINE ( 'NONE', #7886, #18481 ) ;
#6609=ORIENTED_EDGE ( 'NONE', *, *, #6762, .T. ) ;
#6612=VECTOR ( 'NONE', #7457, 1000.000000000000000 ) ;
#6641=EDGE_CURVE ( 'NONE', #8073, #16874, #10391, .T. ) ;
#6643=CARTESIAN_POINT ( 'NONE',  ( -50.00000000000001421, 33.00000000000000000, 44.99999999999999289 ) ) ;
#6648=ORIENTED_EDGE ( 'NONE', *, *, #14320, .F. ) ;
#6653=CARTESIAN_POINT ( 'NONE',  ( 50.00000000000000000, 118.0000000000000142, -60.00000000000000000 ) ) ;
#6656=DIRECTION ( 'NONE',  ( -0.000000000000000000, -0.7071067811865456854, -0.7071067811865494601 ) ) ;
#6658=EDGE_CURVE ( 'NONE', #14054, #15935, #17655, .T. ) ;
#6669=CLOSED_SHELL ( 'NONE', ( #13824, #11391, #3292, #14301, #3077, #5675, #11159, #2071, #10716, #4333, #15355, #15726, #12386, #5481, #17441, #14266, #5830, #12998, #17418, #3038, #1489, #10349, #10471, #13316, #14310, #6419, #9155, #19198, #6523, #13048, #6888, #1217, #16857, #18862, #4448, #11307, #6327, #17665, #102, #18017, #2401, #10217, #17746, #2586, #13047, #1990, #17157, #5119, #9590, #12383 ) ) ;
#6675=DIRECTION ( 'NONE',  ( 0.000000000000000000, 0.000000000000000000, -1.000000000000000000 ) ) ;
#6681=DIRECTION ( 'NONE',  ( 0.000000000000000000, 0.000000000000000000, -1.000000000000000000 ) ) ;
#6685=DIRECTION ( 'NONE',  ( 0.000000000000000000, 0.7071067811865456854, 0.7071067811865494601 ) ) ;
#6724=ORIENTED_EDGE ( 'NONE', *, *, #17019, .T. ) ;
#6726=SURFACE_STYLE_USAGE ( .BOTH. , #3788 ) ;
#6746=VECTOR ( 'NONE', #2629, 1000.000000000000000 ) ;
#6762=EDGE_CURVE ( 'NONE', #6468, #9777, #14918, .T. ) ;
#6789=ORIENTED_EDGE ( 'NONE', *, *, #8293, .F. ) ;
#6798=FACE_OUTER_BOUND ( 'NONE', #11937, .T. ) ;
#6800=ORIENTED_EDGE ( 'NONE', *, *, #5604, .F. ) ;
#6825=DIRECTION ( 'NONE',  ( 1.156482317317871725E-16, 0.000000000000000000, -1.000000000000000000 ) ) ;
#6848=LINE ( 'NONE', #2532, #9700 ) ;
#6863=EDGE_CURVE ( 'NONE', #7196, #17051, #16581, .T. ) ;
#6884=DIRECTION ( 'NONE',  ( 0.000000000000000000, 0.000000000000000000, -1.000000000000000000 ) ) ;
#6888=ADVANCED_FACE ( 'NONE', ( #15212, #12263, #1782, #1683, #3352, #9317 ), #7959, .T. ) ;
#6892=AXIS2_PLACEMENT_3D ( 'NONE', #2131, #8371, #11680 ) ;
#6905=CARTESIAN_POINT ( 'NONE',  ( -45.00000000000000000, 3.000000000000000000, 54.99999999999998579 ) ) ;
#6926=VECTOR ( 'NONE', #8419, 1000.000000000000000 ) ;
#6940=VECTOR ( 'NONE', #8238, 1000.000000000000000 ) ;
#6948=VERTEX_POINT ( 'NONE', #4731 ) ;
#6950=CARTESIAN_POINT ( 'NONE',  ( -1.040834085586084257E-14, 27.62132034355962773, 54.62132034355965260 ) ) ;
#6951=DIRECTION ( 'NONE',  ( 1.000000000000000000, 0.000000000000000000, -4.081702296416016490E-16 ) ) ;
#6953=CARTESIAN_POINT ( 'NONE',  ( -1.040834085586084257E-14, 23.37867965644034030, 50.37867965644033319 ) ) ;
#6974=LINE ( 'NONE', #3939, #5488 ) ;
#7005=( NAMED_UNIT ( * ) SI_UNIT ( $, .STERADIAN. ) SOLID_ANGLE_UNIT ( ) );
#7016=PLANE ( 'NONE',  #14660 ) ;
#7019=AXIS2_PLACEMENT_3D ( 'NONE', #12100, #13670, #1722 ) ;
#7059=VERTEX_POINT ( 'NONE', #17920 ) ;
#7061=VECTOR ( 'NONE', #675, 1000.000000000000000 ) ;
#7067=CARTESIAN_POINT ( 'NONE',  ( -47.00000000000002132, 118.0000000000000142, -60.00000000000002132 ) ) ;
#7079=ORIENTED_EDGE ( 'NONE', *, *, #10487, .T. ) ;
#7080=VECTOR ( 'NONE', #14846, 1000.000000000000000 ) ;
#7126=EDGE_LOOP ( 'NONE', ( #5860, #8497, #18225, #15673 ) ) ;
#7144=LINE ( 'NONE', #8616, #5188 ) ;
#7147=ORIENTED_EDGE ( 'NONE', *, *, #3776, .F. ) ;
#7151=DIRECTION ( 'NONE',  ( -1.000000000000000000, 0.000000000000000000, -1.156482317317871725E-16 ) ) ;
#7155=ORIENTED_EDGE ( 'NONE', *, *, #1203, .T. ) ;
#7173=ORIENTED_EDGE ( 'NONE', *, *, #2198, .T. ) ;
#7196=VERTEX_POINT ( 'NONE', #4654 ) ;
#7210=VECTOR ( 'NONE', #8076, 1000.000000000000000 ) ;
#7222=ORIENTED_EDGE ( 'NONE', *, *, #17739, .T. ) ;
#7235=AXIS2_PLACEMENT_3D ( 'NONE', #17286, #6884, #11379 ) ;
#7257=VERTEX_POINT ( 'NONE', #12183 ) ;
#7259=FACE_OUTER_BOUND ( 'NONE', #8218, .T. ) ;
#7275=DIRECTION ( 'NONE',  ( -0.000000000000000000, -1.000000000000000000, -0.000000000000000000 ) ) ;
#7297=EDGE_LOOP ( 'NONE', ( #8169, #13921, #4317, #16234 ) ) ;
#7305=LINE ( 'NONE', #16331, #15309 ) ;
#7307=CARTESIAN_POINT ( 'NONE',  ( -2.749999999999989786, 38.00000000000000000, -42.68883962248118991 ) ) ;
#7321=VERTEX_POINT ( 'NONE', #2096 ) ;
#7332=VECTOR ( 'NONE', #15832, 1000.000000000000000 ) ;
#7343=STYLED_ITEM ( 'NONE', ( #3974 ), #11772 ) ;
#7355=CARTESIAN_POINT ( 'NONE',  ( -44.99999999999998579, 6.000000000000000000, -56.50000000000000000 ) ) ;
#7356=ORIENTED_EDGE ( 'NONE', *, *, #9841, .F. ) ;
#7408=DIRECTION ( 'NONE',  ( -0.000000000000000000, -1.000000000000000000, -0.000000000000000000 ) ) ;
#7409=LINE ( 'NONE', #7307, #13733 ) ;
#7413=VECTOR ( 'NONE', #19119, 1000.000000000000000 ) ;
#7448=EDGE_CURVE ( 'NONE', #13439, #2933, #1998, .T. ) ;
#7456=ORIENTED_EDGE ( 'NONE', *, *, #12764, .F. ) ;
#7457=DIRECTION ( 'NONE',  ( -0.000000000000000000, 1.000000000000000000, -0.000000000000000000 ) ) ;
#7464=EDGE_CURVE ( 'NONE', #5915, #11555, #431, .T. ) ;
#7465=CARTESIAN_POINT ( 'NONE',  ( -1.040834085586084257E-14, -42.00099999999996214, -15.00100000000031208 ) ) ;
#7500=PLANE ( 'NONE',  #1244 ) ;
#7507=DIRECTION ( 'NONE',  ( 3.826732013112564095E-16, -1.000000000000000000, -1.632680918566406793E-16 ) ) ;
#7509=VECTOR ( 'NONE', #4001, 1000.000000000000000 ) ;
#7534=DIRECTION ( 'NONE',  ( 0.000000000000000000, -0.7071067811865455743, -0.7071067811865495711 ) ) ;
#7539=VECTOR ( 'NONE', #6675, 1000.000000000000000 ) ;
#7541=ORIENTED_EDGE ( 'NONE', *, *, #17150, .F. ) ;
#7547=VERTEX_POINT ( 'NONE', #18852 ) ;
#7552=VERTEX_POINT ( 'NONE', #899 ) ;
#7565=LINE ( 'NONE', #4535, #63 ) ;
#7567=EDGE_CURVE ( 'NONE', #11531, #5928, #15807, .T. ) ;
#7574=ORIENTED_EDGE ( 'NONE', *, *, #17493, .F. ) ;
#7584=ORIENTED_EDGE ( 'NONE', *, *, #17230, .T. ) ;
#7624=EDGE_LOOP ( 'NONE', ( #9776, #16715, #2716, #13193 ) ) ;
#7633=DIRECTION ( 'NONE',  ( 1.000000000000000000, 0.000000000000000000, 0.000000000000000000 ) ) ;
#7644=ORIENTED_EDGE ( 'NONE', *, *, #17150, .T. ) ;
#7646=DIRECTION ( 'NONE',  ( 1.000000000000000000, 0.000000000000000000, 0.000000000000000000 ) ) ;
#7668=AXIS2_PLACEMENT_3D ( 'NONE', #10509, #13357, #1703 ) ;
#7722=( NAMED_UNIT ( * ) PLANE_ANGLE_UNIT ( ) SI_UNIT ( $, .RADIAN. ) );
#7741=VECTOR ( 'NONE', #14643, 1000.000000000000000 ) ;
#7746=ORIENTED_EDGE ( 'NONE', *, *, #15046, .F. ) ;
#7759=ORIENTED_EDGE ( 'NONE', *, *, #16094, .F. ) ;
#7771=CARTESIAN_POINT ( 'NONE',  ( -47.00000000000002132, 30.00000000000000000, -60.00000000000002132 ) ) ;
#7779=CARTESIAN_POINT ( 'NONE',  ( 43.50000000000001421, 118.0000000000000142, 32.49999999999998579 ) ) ;
#7797=DIRECTION ( 'NONE',  ( 0.000000000000000000, 0.000000000000000000, -1.000000000000000000 ) ) ;
#7800=AXIS2_PLACEMENT_3D ( 'NONE', #10263, #7534, #1462 ) ;
#7807=CARTESIAN_POINT ( 'NONE',  ( -50.00000000000002132, 118.0000000000000142, 40.49999999999997868 ) ) ;
#7820=EDGE_LOOP ( 'NONE', ( #17242, #4026, #8172, #3271 ) ) ;
#7859=ORIENTED_EDGE ( 'NONE', *, *, #10439, .F. ) ;
#7872=VECTOR ( 'NONE', #14617, 1000.000000000000000 ) ;
#7878=DIRECTION ( 'NONE',  ( -1.000000000000000000, 0.000000000000000000, -0.000000000000000000 ) ) ;
#7879=ORIENTED_EDGE ( 'NONE', *, *, #3495, .F. ) ;
#7883=LINE ( 'NONE', #425, #7210 ) ;
#7886=CARTESIAN_POINT ( 'NONE',  ( -45.00000000000000000, 3.000000000000000000, 56.49999999999998579 ) ) ;
#7909=CARTESIAN_POINT ( 'NONE',  ( -2.750000000000020872, 118.0000000000000142, 40.49999999999995737 ) ) ;
#7923=ORIENTED_EDGE ( 'NONE', *, *, #476, .T. ) ;
#7947=ORIENTED_EDGE ( 'NONE', *, *, #11613, .F. ) ;
#7959=PLANE ( 'NONE',  #13155 ) ;
#7962=CARTESIAN_POINT ( 'NONE',  ( 44.99999999999998579, 3.000000000000000000, -54.99999999999998579 ) ) ;
#7981=EDGE_LOOP ( 'NONE', ( #796, #18636, #7923, #11233, #12336, #3221, #5752 ) ) ;
#7993=EDGE_LOOP ( 'NONE', ( #17398, #7879, #17509, #14314 ) ) ;
#8028=ORIENTED_EDGE ( 'NONE', *, *, #8229, .T. ) ;
#8029=FACE_OUTER_BOUND ( 'NONE', #4267, .T. ) ;
#8030=DIRECTION ( 'NONE',  ( -1.000000000000000000, 0.000000000000000000, 0.000000000000000000 ) ) ;
#8035=EDGE_CURVE ( 'NONE', #10686, #6595, #8124, .T. ) ;
#8036=LINE ( 'NONE', #11051, #5356 ) ;
#8050=DIRECTION ( 'NONE',  ( -1.000000000000000000, 0.000000000000000000, 0.000000000000000000 ) ) ;
#8053=VECTOR ( 'NONE', #1172, 1000.000000000000000 ) ;
#8060=CARTESIAN_POINT ( 'NONE',  ( -21.50000000000000000, 118.0000000000000142, 32.50000000000000000 ) ) ;
#8069=EDGE_LOOP ( 'NONE', ( #16655, #13413, #8709, #3146 ) ) ;
#8073=VERTEX_POINT ( 'NONE', #3887 ) ;
#8076=DIRECTION ( 'NONE',  ( -1.000000000000000000, 0.000000000000000000, -0.000000000000000000 ) ) ;
#8080=DIRECTION ( 'NONE',  ( 0.000000000000000000, -1.000000000000000000, 0.000000000000000000 ) ) ;
#8098=LINE ( 'NONE', #10923, #289 ) ;
#8119=VECTOR ( 'NONE', #13873, 1000.000000000000000 ) ;
#8124=LINE ( 'NONE', #14096, #16002 ) ;
#8128=CARTESIAN_POINT ( 'NONE',  ( 50.00000000000000000, 3.000000000000000000, -60.00000000000000000 ) ) ;
#8129=ORIENTED_EDGE ( 'NONE', *, *, #17399, .F. ) ;
#8144=AXIS2_PLACEMENT_3D ( 'NONE', #8825, #3040, #14810 ) ;
#8159=ORIENTED_EDGE ( 'NONE', *, *, #6526, .F. ) ;
#8169=ORIENTED_EDGE ( 'NONE', *, *, #9778, .F. ) ;
#8172=ORIENTED_EDGE ( 'NONE', *, *, #757, .F. ) ;
#8173=CARTESIAN_POINT ( 'NONE',  ( -47.00000000000002132, 115.0000000000000000, -57.00000000000001421 ) ) ;
#8193=VECTOR ( 'NONE', #5208, 1000.000000000000000 ) ;
#8208=VECTOR ( 'NONE', #15680, 1000.000000000000000 ) ;
#8210=EDGE_CURVE ( 'NONE', #5477, #7059, #8679, .T. ) ;
#8218=EDGE_LOOP ( 'NONE', ( #1045, #3244, #871, #13019 ) ) ;
#8229=EDGE_CURVE ( 'NONE', #2670, #4095, #11933, .T. ) ;
#8238=DIRECTION ( 'NONE',  ( -0.000000000000000000, -1.000000000000000000, -0.000000000000000000 ) ) ;
#8247=DIRECTION ( 'NONE',  ( 1.000000000000000000, 0.000000000000000000, 0.000000000000000000 ) ) ;
#8249=DIRECTION ( 'NONE',  ( 0.000000000000000000, 1.632680918566406793E-16, -1.000000000000000000 ) ) ;
#8291=AXIS2_PLACEMENT_3D ( 'NONE', #18096, #16523, #10530 ) ;
#8293=EDGE_CURVE ( 'NONE', #13385, #11368, #19374, .T. ) ;
#8315=AXIS2_PLACEMENT_3D ( 'NONE', #17170, #15882, #14403 ) ;
#8318=VECTOR ( 'NONE', #3691, 1000.000000000000000 ) ;
#8338=FACE_OUTER_BOUND ( 'NONE', #6182, .T. ) ;
#8347=VECTOR ( 'NONE', #7878, 1000.000000000000000 ) ;
#8348=AXIS2_PLACEMENT_3D ( 'NONE', #16990, #6685, #3450 ) ;
#8349=DIRECTION ( 'NONE',  ( -1.000000000000000000, 0.000000000000000000, 0.000000000000000000 ) ) ;
#8350=VERTEX_POINT ( 'NONE', #4579 ) ;
#8362=EDGE_CURVE ( 'NONE', #12628, #16874, #18404, .T. ) ;
#8371=DIRECTION ( 'NONE',  ( -0.000000000000000000, 0.7071067811865456854, 0.7071067811865494601 ) ) ;
#8379=DIRECTION ( 'NONE',  ( 1.000000000000000000, -0.000000000000000000, -0.000000000000000000 ) ) ;
#8409=CIRCLE ( 'NONE', #10913, 10.00000000000000178 ) ;
#8410=CARTESIAN_POINT ( 'NONE',  ( 44.99999999999998579, 3.000000000000000000, -54.99999999999998579 ) ) ;
#8412=CARTESIAN_POINT ( 'NONE',  ( 43.49999999999997868, 2.999000000000001442, -52.50000000000002132 ) ) ;
#8419=DIRECTION ( 'NONE',  ( 1.000000000000000000, -0.000000000000000000, -0.000000000000000000 ) ) ;
#8447=DIRECTION ( 'NONE',  ( 0.000000000000000000, -1.000000000000000000, 0.000000000000000000 ) ) ;
#8497=ORIENTED_EDGE ( 'NONE', *, *, #13961, .T. ) ;
#8527=VERTEX_POINT ( 'NONE', #644 ) ;
#8541=LINE ( 'NONE', #896, #322 ) ;
#8543=CARTESIAN_POINT ( 'NONE',  ( -1.040834085586084257E-14, 32.57106781186547551, 49.67157287525382969 ) ) ;
#8544=DIRECTION ( 'NONE',  ( 1.156482317317871725E-16, 0.000000000000000000, -1.000000000000000000 ) ) ;
#8552=ORIENTED_EDGE ( 'NONE', *, *, #1109, .F. ) ;
#8574=AXIS2_PLACEMENT_3D ( 'NONE', #6323, #339, #6515 ) ;
#8585=( GEOMETRIC_REPRESENTATION_CONTEXT ( 3 ) GLOBAL_UNCERTAINTY_ASSIGNED_CONTEXT ( ( #9037 ) ) GLOBAL_UNIT_ASSIGNED_CONTEXT ( ( #653, #1031, #7005 ) ) REPRESENTATION_CONTEXT ( 'NONE', 'WORKASPACE' ) );
#8589=DIRECTION ( 'NONE',  ( 3.826732013112564095E-16, -1.000000000000000000, -1.632680918566406793E-16 ) ) ;
#8591=ORIENTED_EDGE ( 'NONE', *, *, #17392, .T. ) ;
#8608=LINE ( 'NONE', #11252, #6926 ) ;
#8609=LINE ( 'NONE', #1162, #2467 ) ;
#8616=CARTESIAN_POINT ( 'NONE',  ( 50.00000000000000000, 33.00000000000000000, 59.99999999999997868 ) ) ;
#8617=ORIENTED_EDGE ( 'NONE', *, *, #3495, .T. ) ;
#8622=EDGE_LOOP ( 'NONE', ( #14812, #14683, #17946, #1371 ) ) ;
#8656=DIRECTION ( 'NONE',  ( 8.163404592832032733E-17, 0.000000000000000000, 1.000000000000000000 ) ) ;
#8658=DIRECTION ( 'NONE',  ( 0.000000000000000000, 0.7071067811865456854, 0.7071067811865494601 ) ) ;
#8660=AXIS2_PLACEMENT_3D ( 'NONE', #4168, #10119, #13167 ) ;
#8679=LINE ( 'NONE', #1436, #2865 ) ;
#8681=CARTESIAN_POINT ( 'NONE',  ( 50.00000000000000000, 6.000000000000005329, -56.99999999999999289 ) ) ;
#8682=LINE ( 'NONE', #13085, #10513 ) ;
#8690=EDGE_CURVE ( 'NONE', #18230, #5758, #8728, .T. ) ;
#8693=DIRECTION ( 'NONE',  ( -1.000000000000000000, -3.826732013112563602E-16, 0.000000000000000000 ) ) ;
#8707=VERTEX_POINT ( 'NONE', #13037 ) ;
#8709=ORIENTED_EDGE ( 'NONE', *, *, #12707, .T. ) ;
#8714=ORIENTED_EDGE ( 'NONE', *, *, #11090, .T. ) ;
#8723=ORIENTED_EDGE ( 'NONE', *, *, #2292, .T. ) ;
#8728=LINE ( 'NONE', #17118, #14436 ) ;
#8749=CARTESIAN_POINT ( 'NONE',  ( 44.99999999999998579, 3.000000000000000000, -54.99999999999998579 ) ) ;
#8768=AXIS2_PLACEMENT_3D ( 'NONE', #6953, #3124, #14245 ) ;
#8803=ORIENTED_EDGE ( 'NONE', *, *, #9256, .T. ) ;
#8820=CIRCLE ( 'NONE', #11316, 1.500000000000001332 ) ;
#8825=CARTESIAN_POINT ( 'NONE',  ( -50.00000000000002132, 33.00000000000000000, 44.99999999999999289 ) ) ;
#8836=EDGE_CURVE ( 'NONE', #13043, #3590, #12161, .T. ) ;
#8842=ORIENTED_EDGE ( 'NONE', *, *, #11284, .F. ) ;
#8862=ORIENTED_EDGE ( 'NONE', *, *, #4967, .T. ) ;
#8871=EDGE_CURVE ( 'NONE', #18238, #8707, #7565, .T. ) ;
#8896=CARTESIAN_POINT ( 'NONE',  ( 41.99999999999998579, 139.6861997365471950, -52.00000000000000000 ) ) ;
#8932=DIRECTION ( 'NONE',  ( 0.000000000000000000, -0.7071067811865495711, 0.7071067811865454633 ) ) ;
#8935=ORIENTED_EDGE ( 'NONE', *, *, #12424, .F. ) ;
#8944=DIRECTION ( 'NONE',  ( 0.000000000000000000, 0.000000000000000000, -1.000000000000000000 ) ) ;
#8949=DIRECTION ( 'NONE',  ( 0.000000000000000000, -0.7071067811865492381, 0.7071067811865456854 ) ) ;
#8953=CIRCLE ( 'NONE', #12699, 6.000000000000003553 ) ;
#8959=EDGE_LOOP ( 'NONE', ( #4826, #5662 ) ) ;
#8973=DIRECTION ( 'NONE',  ( 0.000000000000000000, -1.000000000000000000, 0.000000000000000000 ) ) ;
#9008=VERTEX_POINT ( 'NONE', #1982 ) ;
#9037=UNCERTAINTY_MEASURE_WITH_UNIT (LENGTH_MEASURE( 1.000000000000000082E-05 ), #653, 'distance_accuracy_value', 'NONE');
#9045=ORIENTED_EDGE ( 'NONE', *, *, #17392, .F. ) ;
#9049=DIRECTION ( 'NONE',  ( -0.000000000000000000, -1.000000000000000000, -0.000000000000000000 ) ) ;
#9099=VECTOR ( 'NONE', #9127, 1000.000000000000000 ) ;
#9122=CARTESIAN_POINT ( 'NONE',  ( -50.00000000000002132, 33.00000000000000000, 40.49999999999996447 ) ) ;
#9127=DIRECTION ( 'NONE',  ( 1.000000000000000000, -0.000000000000000000, 0.000000000000000000 ) ) ;
#9144=CIRCLE ( 'NONE', #10378, 1.500000000000001332 ) ;
#9149=FACE_OUTER_BOUND ( 'NONE', #12753, .T. ) ;
#9155=ADVANCED_FACE ( 'NONE', ( #8338 ), #17537, .T. ) ;
#9174=CARTESIAN_POINT ( 'NONE',  ( 2.750000000000009326, 37.99999999999999289, 37.49999999999996447 ) ) ;
#9186=ORIENTED_EDGE ( 'NONE', *, *, #5234, .F. ) ;
#9222=DIRECTION ( 'NONE',  ( 0.000000000000000000, 0.000000000000000000, -1.000000000000000000 ) ) ;
#9225=DIRECTION ( 'NONE',  ( -0.000000000000000000, -0.7071067811865456854, -0.7071067811865493491 ) ) ;
#9246=DIRECTION ( 'NONE',  ( -0.000000000000000000, -0.000000000000000000, 1.000000000000000000 ) ) ;
#9248=CARTESIAN_POINT ( 'NONE',  ( 44.99999999999998579, 6.000000000000000000, -53.49999999999998579 ) ) ;
#9256=EDGE_CURVE ( 'NONE', #2227, #13385, #16067, .T. ) ;
#9265=LINE ( 'NONE', #12202, #11222 ) ;
#9273=DIRECTION ( 'NONE',  ( 1.000000000000000000, -0.000000000000000000, 0.000000000000000000 ) ) ;
#9300=EDGE_LOOP ( 'NONE', ( #17041, #5965, #4757, #13823 ) ) ;
#9317=FACE_OUTER_BOUND ( 'NONE', #8069, .T. ) ;
#9319=CARTESIAN_POINT ( 'NONE',  ( 44.99999999999997158, 3.000000000000000000, 55.00000000000000000 ) ) ;
#9333=ORIENTED_EDGE ( 'NONE', *, *, #8035, .F. ) ;
#9338=DIRECTION ( 'NONE',  ( 1.000000000000000000, 0.000000000000000000, 0.000000000000000000 ) ) ;
#9348=EDGE_CURVE ( 'NONE', #15084, #2159, #1598, .T. ) ;
#9350=CARTESIAN_POINT ( 'NONE',  ( -1.040834085586084257E-14, 32.57106781186547551, 49.67157287525382969 ) ) ;
#9353=CARTESIAN_POINT ( 'NONE',  ( -43.50000000000000000, 2.999000000000001442, 32.50000000000000000 ) ) ;
#9368=VECTOR ( 'NONE', #8080, 1000.000000000000000 ) ;
#9413=CARTESIAN_POINT ( 'NONE',  ( 0.000000000000000000, 6.000000000000000000, 0.000000000000000000 ) ) ;
#9417=FACE_OUTER_BOUND ( 'NONE', #2964, .T. ) ;
#9421=DIRECTION ( 'NONE',  ( -0.000000000000000000, -1.000000000000000000, -0.000000000000000000 ) ) ;
#9428=VECTOR ( 'NONE', #2413, 1000.000000000000000 ) ;
#9456=LINE ( 'NONE', #9547, #2884 ) ;
#9511=DIRECTION ( 'NONE',  ( 0.000000000000000000, 1.000000000000000000, 1.632680918566406793E-16 ) ) ;
#9533=CYLINDRICAL_SURFACE ( 'NONE', #11416, 7.000000000000001776 ) ;
#9535=CIRCLE ( 'NONE', #11100, 1.500000000000001332 ) ;
#9538=DIRECTION ( 'NONE',  ( 0.000000000000000000, 1.000000000000000000, 0.000000000000000000 ) ) ;
#9547=CARTESIAN_POINT ( 'NONE',  ( 44.99999999999998579, 3.000000000000000000, -56.49999999999998579 ) ) ;
#9571=ORIENTED_EDGE ( 'NONE', *, *, #4104, .F. ) ;
#9590=ADVANCED_FACE ( 'NONE', ( #13806 ), #4996, .T. ) ;
#9599=AXIS2_PLACEMENT_3D ( 'NONE', #16468, #7151, #4416 ) ;
#9603=CARTESIAN_POINT ( 'NONE',  ( -43.50000000000000000, 115.0000000000000000, 32.50000000000000000 ) ) ;
#9613=DIRECTION ( 'NONE',  ( 4.898042755699219393E-16, 0.000000000000000000, 1.000000000000000000 ) ) ;
#9619=ORIENTED_EDGE ( 'NONE', *, *, #2516, .T. ) ;
#9621=EDGE_CURVE ( 'NONE', #14552, #7196, #8036, .T. ) ;
#9625=LINE ( 'NONE', #15610, #923 ) ;
#9651=DIRECTION ( 'NONE',  ( 0.000000000000000000, 0.000000000000000000, -1.000000000000000000 ) ) ;
#9674=DIRECTION ( 'NONE',  ( 0.000000000000000000, 0.7071067811865494601, -0.7071067811865456854 ) ) ;
#9675=VECTOR ( 'NONE', #11833, 1000.000000000000000 ) ;
#9677=ORIENTED_EDGE ( 'NONE', *, *, #12084, .F. ) ;
#9683=VERTEX_POINT ( 'NONE', #1954 ) ;
#9687=CARTESIAN_POINT ( 'NONE',  ( -50.00000000000002132, 30.00000000000000355, 37.49999999999996447 ) ) ;
#9693=CARTESIAN_POINT ( 'NONE',  ( 44.99999999999998579, 6.000000000000000000, -56.49999999999998579 ) ) ;
#9698=DIRECTION ( 'NONE',  ( 0.000000000000000000, 0.7071067811865456854, 0.7071067811865493491 ) ) ;
#9700=VECTOR ( 'NONE', #18639, 1000.000000000000114 ) ;
#9726=AXIS2_PLACEMENT_3D ( 'NONE', #1852, #6656, #9674 ) ;
#9744=FACE_OUTER_BOUND ( 'NONE', #6272, .T. ) ;
#9753=CARTESIAN_POINT ( 'NONE',  ( -9.673552776372430100E-15, 27.62132034355963839, 46.13603896932106352 ) ) ;
#9755=EDGE_LOOP ( 'NONE', ( #122, #7947, #10568, #14285 ) ) ;
#9772=ORIENTED_EDGE ( 'NONE', *, *, #14705, .F. ) ;
#9776=ORIENTED_EDGE ( 'NONE', *, *, #4394, .T. ) ;
#9777=VERTEX_POINT ( 'NONE', #5373 ) ;
#9778=EDGE_CURVE ( 'NONE', #8350, #14552, #11229, .T. ) ;
#9784=ORIENTED_EDGE ( 'NONE', *, *, #10324, .T. ) ;
#9797=DIRECTION ( 'NONE',  ( -1.000000000000000000, 0.000000000000000000, 4.898042755699219393E-16 ) ) ;
#9841=EDGE_CURVE ( 'NONE', #10684, #11368, #3889, .T. ) ;
#9852=VECTOR ( 'NONE', #10093, 1000.000000000000000 ) ;
#9854=DIRECTION ( 'NONE',  ( 0.000000000000000000, -0.7071067811865455743, -0.7071067811865495711 ) ) ;
#9878=CARTESIAN_POINT ( 'NONE',  ( -43.50000000000000000, 2.999000000000001442, 32.50000000000000000 ) ) ;
#9889=FACE_OUTER_BOUND ( 'NONE', #4028, .T. ) ;
#9909=LINE ( 'NONE', #12856, #15797 ) ;
#9920=DIRECTION ( 'NONE',  ( 0.000000000000000000, 0.000000000000000000, -1.000000000000000000 ) ) ;
#9989=LINE ( 'NONE', #16081, #1287 ) ;
#9998=AXIS2_PLACEMENT_3D ( 'NONE', #17431, #10062, #11345 ) ;
#10020=AXIS2_PLACEMENT_3D ( 'NONE', #11355, #2538, #11540 ) ;
#10025=VECTOR ( 'NONE', #3143, 1000.000000000000000 ) ;
#10029=VECTOR ( 'NONE', #14238, 1000.000000000000000 ) ;
#10039=VECTOR ( 'NONE', #6262, 1000.000000000000000 ) ;
#10062=DIRECTION ( 'NONE',  ( 0.000000000000000000, 0.7071067811865456854, 0.7071067811865494601 ) ) ;
#10065=LINE ( 'NONE', #18635, #7539 ) ;
#10093=DIRECTION ( 'NONE',  ( 1.000000000000000000, 0.000000000000000000, 0.000000000000000000 ) ) ;
#10106=EDGE_CURVE ( 'NONE', #11279, #11949, #17009, .T. ) ;
#10119=DIRECTION ( 'NONE',  ( -0.000000000000000000, -1.000000000000000000, -0.000000000000000000 ) ) ;
#10155=DIRECTION ( 'NONE',  ( 0.000000000000000000, 0.000000000000000000, -1.000000000000000000 ) ) ;
#10166=CARTESIAN_POINT ( 'NONE',  ( 44.99999999999997158, 3.000000000000000000, 55.00000000000000000 ) ) ;
#10175=VERTEX_POINT ( 'NONE', #15141 ) ;
#10178=DIRECTION ( 'NONE',  ( -1.888166612144349831E-32, 1.000000000000000000, 1.632680918566406793E-16 ) ) ;
#10190=DIRECTION ( 'NONE',  ( 3.826732013112563602E-16, -1.000000000000000000, 0.000000000000000000 ) ) ;
#10212=CARTESIAN_POINT ( 'NONE',  ( 0.000000000000000000, 3.000000000000000000, 51.99999999999997868 ) ) ;
#10217=ADVANCED_FACE ( 'NONE', ( #18944 ), #15619, .T. ) ;
#10218=CIRCLE ( 'NONE', #8660, 1.500000000000001332 ) ;
#10223=LINE ( 'NONE', #10318, #4203 ) ;
#10241=CYLINDRICAL_SURFACE ( 'NONE', #3713, 1.500000000000001332 ) ;
#10250=ORIENTED_EDGE ( 'NONE', *, *, #5789, .T. ) ;
#10263=CARTESIAN_POINT ( 'NONE',  ( -1.040834085586084257E-14, 25.49999999999996803, 52.49999999999998579 ) ) ;
#10272=VECTOR ( 'NONE', #17303, 1000.000000000000000 ) ;
#10311=DIRECTION ( 'NONE',  ( 0.000000000000000000, 0.000000000000000000, -1.000000000000000000 ) ) ;
#10318=CARTESIAN_POINT ( 'NONE',  ( -43.50000000000000711, 2.999000000000001442, -52.50000000000000711 ) ) ;
#10322=ORIENTED_EDGE ( 'NONE', *, *, #476, .F. ) ;
#10324=EDGE_CURVE ( 'NONE', #2359, #5477, #3540, .T. ) ;
#10344=DIRECTION ( 'NONE',  ( -0.000000000000000000, 1.000000000000000000, -0.000000000000000000 ) ) ;
#10349=ADVANCED_FACE ( 'NONE', ( #15407 ), #5118, .F. ) ;
#10350=VECTOR ( 'NONE', #7633, 1000.000000000000000 ) ;
#10378=AXIS2_PLACEMENT_3D ( 'NONE', #4781, #13775, #17630 ) ;
#10385=EDGE_CURVE ( 'NONE', #8527, #3207, #17071, .T. ) ;
#10389=DIRECTION ( 'NONE',  ( -0.000000000000000000, -0.7071067811865456854, -0.7071067811865494601 ) ) ;
#10391=LINE ( 'NONE', #5600, #7872 ) ;
#10400=CARTESIAN_POINT ( 'NONE',  ( 49.99999999999998579, 118.0000000000000142, 40.49999999999997868 ) ) ;
#10417=FACE_OUTER_BOUND ( 'NONE', #16659, .T. ) ;
#10434=FACE_OUTER_BOUND ( 'NONE', #17972, .T. ) ;
#10439=EDGE_CURVE ( 'NONE', #12326, #15077, #5017, .T. ) ;
#10458=FACE_OUTER_BOUND ( 'NONE', #458, .T. ) ;
#10471=ADVANCED_FACE ( 'NONE', ( #12734 ), #18914, .F. ) ;
#10487=EDGE_CURVE ( 'NONE', #4412, #18230, #8608, .T. ) ;
#10490=AXIS2_PLACEMENT_3D ( 'NONE', #5583, #9797, #9613 ) ;
#10504=DIRECTION ( 'NONE',  ( 0.000000000000000000, 0.000000000000000000, -1.000000000000000000 ) ) ;
#10509=CARTESIAN_POINT ( 'NONE',  ( 44.99999999999997158, 3.000000000000000000, 55.00000000000000000 ) ) ;
#10513=VECTOR ( 'NONE', #10344, 1000.000000000000000 ) ;
#10530=DIRECTION ( 'NONE',  ( 0.000000000000000000, 0.000000000000000000, -1.000000000000000000 ) ) ;
#10559=DIRECTION ( 'NONE',  ( -6.672013369141567928E-17, 0.000000000000000000, 1.000000000000000000 ) ) ;
#10568=ORIENTED_EDGE ( 'NONE', *, *, #16748, .T. ) ;
#10577=CARTESIAN_POINT ( 'NONE',  ( -1.040834085586084257E-14, 30.44974746830581580, 47.55025253169416288 ) ) ;
#10604=ORIENTED_EDGE ( 'NONE', *, *, #16680, .F. ) ;
#10627=VECTOR ( 'NONE', #3145, 1000.000000000000000 ) ;
#10656=VECTOR ( 'NONE', #2751, 1000.000000000000000 ) ;
#10667=ORIENTED_EDGE ( 'NONE', *, *, #10324, .F. ) ;
#10674=EDGE_CURVE ( 'NONE', #2933, #5783, #9144, .T. ) ;
#10684=VERTEX_POINT ( 'NONE', #7909 ) ;
#10685=CARTESIAN_POINT ( 'NONE',  ( -1.040834085586084257E-14, 21.25735931288069125, 56.74264068711926967 ) ) ;
#10686=VERTEX_POINT ( 'NONE', #2729 ) ;
#10716=ADVANCED_FACE ( 'NONE', ( #15156, #14793, #3388, #13874, #13574, #155 ), #11639, .F. ) ;
#10760=EDGE_LOOP ( 'NONE', ( #12315, #7456 ) ) ;
#10777=CARTESIAN_POINT ( 'NONE',  ( -50.00000000000001421, 6.000000000000005329, 56.99999999999997158 ) ) ;
#10804=VERTEX_POINT ( 'NONE', #16124 ) ;
#10829=CARTESIAN_POINT ( 'NONE',  ( 0.000000000000000000, 3.000000000000000000, 0.000000000000000000 ) ) ;
#10856=ORIENTED_EDGE ( 'NONE', *, *, #3059, .F. ) ;
#10878=CARTESIAN_POINT ( 'NONE',  ( -43.50000000000000000, 118.0000000000000142, 32.50000000000000000 ) ) ;
#10904=CARTESIAN_POINT ( 'NONE',  ( 2.749999999999979128, 118.0000000000000142, 40.49999999999995737 ) ) ;
#10905=AXIS2_PLACEMENT_3D ( 'NONE', #15350, #451, #9651 ) ;
#10913=AXIS2_PLACEMENT_3D ( 'NONE', #18001, #6045, #15058 ) ;
#10918=DIRECTION ( 'NONE',  ( -0.000000000000000000, -1.000000000000000000, -0.000000000000000000 ) ) ;
#10923=CARTESIAN_POINT ( 'NONE',  ( 47.00000000000000000, 118.0000000000000142, -56.99999999999999289 ) ) ;
#10948=DIRECTION ( 'NONE',  ( 0.000000000000000000, 1.632680918566406793E-16, -1.000000000000000000 ) ) ;
#10963=ORIENTED_EDGE ( 'NONE', *, *, #17399, .T. ) ;
#10998=ORIENTED_EDGE ( 'NONE', *, *, #805, .F. ) ;
#11002=PLANE ( 'NONE',  #2187 ) ;
#11003=FACE_OUTER_BOUND ( 'NONE', #4740, .T. ) ;
#11028=EDGE_CURVE ( 'NONE', #1710, #15097, #862, .T. ) ;
#11029=EDGE_CURVE ( 'NONE', #18716, #6167, #14205, .T. ) ;
#11047=PLANE ( 'NONE',  #283 ) ;
#11051=CARTESIAN_POINT ( 'NONE',  ( -47.00000000000002132, 6.000000000000005329, -60.00000000000002132 ) ) ;
#11052=CARTESIAN_POINT ( 'NONE',  ( 50.00000000000000000, 33.00000000000000000, 40.49999999999996447 ) ) ;
#11059=ORIENTED_EDGE ( 'NONE', *, *, #14543, .F. ) ;
#11062=DIRECTION ( 'NONE',  ( 1.156482317317871725E-16, 0.000000000000000000, -1.000000000000000000 ) ) ;
#11068=EDGE_LOOP ( 'NONE', ( #12319, #6581, #15321, #10856 ) ) ;
#11072=ORIENTED_EDGE ( 'NONE', *, *, #15388, .F. ) ;
#11073=DIRECTION ( 'NONE',  ( 0.000000000000000000, 0.000000000000000000, -1.000000000000000000 ) ) ;
#11074=LINE ( 'NONE', #15409, #5032 ) ;
#11081=CARTESIAN_POINT ( 'NONE',  ( -45.00000000000000000, 3.000000000000000000, 53.49999999999998579 ) ) ;
#11090=EDGE_CURVE ( 'NONE', #12326, #5758, #12541, .T. ) ;
#11094=CARTESIAN_POINT ( 'NONE',  ( 43.50000000000001421, 118.0000000000000142, 32.49999999999998579 ) ) ;
#11100=AXIS2_PLACEMENT_3D ( 'NONE', #133, #9049, #10311 ) ;
#11103=FACE_BOUND ( 'NONE', #4453, .T. ) ;
#11105=ORIENTED_EDGE ( 'NONE', *, *, #18144, .F. ) ;
#11116=DIRECTION ( 'NONE',  ( 0.000000000000000000, -1.000000000000000000, 0.000000000000000000 ) ) ;
#11120=AXIS2_PLACEMENT_3D ( 'NONE', #7465, #4440, #8932 ) ;
#11126=VERTEX_POINT ( 'NONE', #4750 ) ;
#11136=ORIENTED_EDGE ( 'NONE', *, *, #5325, .T. ) ;
#11138=DIRECTION ( 'NONE',  ( -0.000000000000000000, -1.000000000000000000, -0.000000000000000000 ) ) ;
#11150=EDGE_LOOP ( 'NONE', ( #11059, #13904, #3527, #14488 ) ) ;
#11154=CARTESIAN_POINT ( 'NONE',  ( 49.99999999999998579, 118.0000000000000142, 59.99999999999997868 ) ) ;
#11159=ADVANCED_FACE ( 'NONE', ( #2614 ), #19194, .F. ) ;
#11166=CARTESIAN_POINT ( 'NONE',  ( -45.00000000000000000, 6.000000000000000000, 54.99999999999998579 ) ) ;
#11186=EDGE_LOOP ( 'NONE', ( #16263, #7079, #14155, #15197 ) ) ;
#11211=VECTOR ( 'NONE', #2507, 1000.000000000000114 ) ;
#11222=VECTOR ( 'NONE', #13774, 1000.000000000000000 ) ;
#11223=LINE ( 'NONE', #15659, #15341 ) ;
#11229=LINE ( 'NONE', #8681, #3787 ) ;
#11233=ORIENTED_EDGE ( 'NONE', *, *, #744, .T. ) ;
#11252=CARTESIAN_POINT ( 'NONE',  ( -50.00000000000002132, 30.00000000000000355, 43.75735931288070191 ) ) ;
#11267=EDGE_CURVE ( 'NONE', #7547, #4041, #8820, .T. ) ;
#11268=DIRECTION ( 'NONE',  ( 0.000000000000000000, -0.7071067811865455743, -0.7071067811865495711 ) ) ;
#11279=VERTEX_POINT ( 'NONE', #1153 ) ;
#11284=EDGE_CURVE ( 'NONE', #4512, #7552, #19002, .T. ) ;
#11302=VECTOR ( 'NONE', #6825, 1000.000000000000000 ) ;
#11305=CARTESIAN_POINT ( 'NONE',  ( -2.749999999999989786, 38.00000000000000000, 37.49999999999995737 ) ) ;
#11307=ADVANCED_FACE ( 'NONE', ( #14385 ), #4197, .F. ) ;
#11312=CARTESIAN_POINT ( 'NONE',  ( -47.00000000000002132, 118.0000000000000142, -57.00000000000001421 ) ) ;
#11316=AXIS2_PLACEMENT_3D ( 'NONE', #8410, #13001, #3999 ) ;
#11324=ORIENTED_EDGE ( 'NONE', *, *, #12135, .T. ) ;
#11335=EDGE_LOOP ( 'NONE', ( #6567, #15263, #16343, #6800 ) ) ;
#11340=ORIENTED_EDGE ( 'NONE', *, *, #8362, .T. ) ;
#11345=DIRECTION ( 'NONE',  ( 0.000000000000000000, -0.7071067811865492381, 0.7071067811865457964 ) ) ;
#11349=DIRECTION ( 'NONE',  ( 0.000000000000000000, 0.000000000000000000, -1.000000000000000000 ) ) ;
#11355=CARTESIAN_POINT ( 'NONE',  ( -50.00000000000001421, 118.0000000000000142, 56.99999999999997158 ) ) ;
#11361=DIRECTION ( 'NONE',  ( -3.826732013112564095E-16, 1.000000000000000000, 1.632680918566406793E-16 ) ) ;
#11368=VERTEX_POINT ( 'NONE', #13593 ) ;
#11372=EDGE_CURVE ( 'NONE', #14646, #9008, #4142, .T. ) ;
#11374=CARTESIAN_POINT ( 'NONE',  ( 50.00000000000000000, 118.0000000000000142, 40.49999999999997868 ) ) ;
#11379=DIRECTION ( 'NONE',  ( -1.000000000000000000, 0.000000000000000000, -0.000000000000000000 ) ) ;
#11384=UNCERTAINTY_MEASURE_WITH_UNIT (LENGTH_MEASURE( 1.000000000000000082E-05 ), #403, 'distance_accuracy_value', 'NONE');
#11391=ADVANCED_FACE ( 'NONE', ( #269 ), #12222, .T. ) ;
#11400=CARTESIAN_POINT ( 'NONE',  ( -47.00000000000001421, 115.0000000000000000, 37.49999999999997868 ) ) ;
#11406=EDGE_CURVE ( 'NONE', #12225, #14571, #11998, .T. ) ;
#11416=AXIS2_PLACEMENT_3D ( 'NONE', #12579, #15613, #1997 ) ;
#11423=ORIENTED_EDGE ( 'NONE', *, *, #5992, .F. ) ;
#11437=LINE ( 'NONE', #2616, #14384 ) ;
#11444=FACE_BOUND ( 'NONE', #6478, .T. ) ;
#11456=LINE ( 'NONE', #17448, #13340 ) ;
#11459=AXIS2_PLACEMENT_3D ( 'NONE', #12746, #11268, #18741 ) ;
#11511=EDGE_CURVE ( 'NONE', #4095, #7547, #9456, .T. ) ;
#11521=EDGE_LOOP ( 'NONE', ( #14788, #18484 ) ) ;
#11531=VERTEX_POINT ( 'NONE', #9350 ) ;
#11540=DIRECTION ( 'NONE',  ( -1.000000000000000000, 0.000000000000000000, -0.000000000000000000 ) ) ;
#11555=VERTEX_POINT ( 'NONE', #3769 ) ;
#11557=VECTOR ( 'NONE', #2434, 1000.000000000000000 ) ;
#11564=CARTESIAN_POINT ( 'NONE',  ( -50.00000000000002132, 33.00000000000000000, 44.99999999999999289 ) ) ;
#11604=AXIS2_PLACEMENT_3D ( 'NONE', #17320, #12893, #18893 ) ;
#11613=EDGE_CURVE ( 'NONE', #3909, #13439, #3829, .T. ) ;
#11639=PLANE ( 'NONE',  #15100 ) ;
#11680=DIRECTION ( 'NONE',  ( 0.000000000000000000, -0.7071067811865495711, 0.7071067811865454633 ) ) ;
#11686=CARTESIAN_POINT ( 'NONE',  ( -1.040834085586084257E-14, 25.49999999999998934, 52.50000000000000000 ) ) ;
#11707=FACE_BOUND ( 'NONE', #18806, .T. ) ;
#11710=VECTOR ( 'NONE', #14737, 1000.000000000000000 ) ;
#11713=CARTESIAN_POINT ( 'NONE',  ( -2.750000000000020872, 118.0000000000000000, 37.49999999999997158 ) ) ;
#11724=DIRECTION ( 'NONE',  ( 0.000000000000000000, 0.000000000000000000, -1.000000000000000000 ) ) ;
#11727=EDGE_LOOP ( 'NONE', ( #14526, #168, #2380, #18911, #11105 ) ) ;
#11735=CARTESIAN_POINT ( 'NONE',  ( 2.750000000000009770, 38.00000000000000000, -42.68883962248118991 ) ) ;
#11741=ORIENTED_EDGE ( 'NONE', *, *, #3846, .F. ) ;
#11767=EDGE_CURVE ( 'NONE', #9777, #11949, #5525, .T. ) ;
#11772=ADVANCED_BREP_SHAPE_REPRESENTATION ( '', ( #4051, #1791 ), #15487 ) ;
#11782=DIRECTION ( 'NONE',  ( -0.000000000000000000, -1.000000000000000000, -0.000000000000000000 ) ) ;
#11803=CARTESIAN_POINT ( 'NONE',  ( -41.99999999999997868, 6.000000000000005329, 51.99999999999997868 ) ) ;
#11809=CARTESIAN_POINT ( 'NONE',  ( 46.99999999999998579, 118.0000000000000142, 56.99999999999997158 ) ) ;
#11828=VECTOR ( 'NONE', #8973, 1000.000000000000000 ) ;
#11833=DIRECTION ( 'NONE',  ( 6.672013369141567928E-17, 0.000000000000000000, -1.000000000000000000 ) ) ;
#11837=DIRECTION ( 'NONE',  ( 0.000000000000000000, -0.000000000000000000, 1.000000000000000000 ) ) ;
#11847=CARTESIAN_POINT ( 'NONE',  ( 50.00000000000000000, 118.0000000000000142, -60.00000000000000000 ) ) ;
#11854=DIRECTION ( 'NONE',  ( -5.782411586589357392E-17, 0.000000000000000000, -1.000000000000000000 ) ) ;
#11868=EDGE_CURVE ( 'NONE', #5783, #2933, #17498, .T. ) ;
#11883=EDGE_LOOP ( 'NONE', ( #13907, #11981 ) ) ;
#11909=DIRECTION ( 'NONE',  ( 1.000000000000000000, 0.000000000000000000, -0.000000000000000000 ) ) ;
#11931=CARTESIAN_POINT ( 'NONE',  ( -44.99999999999998579, 6.000000000000000000, -55.00000000000000000 ) ) ;
#11933=CIRCLE ( 'NONE', #13835, 1.500000000000001332 ) ;
#11937=EDGE_LOOP ( 'NONE', ( #13204, #9784, #17617, #18901, #4695, #14908, #2429, #9619 ) ) ;
#11949=VERTEX_POINT ( 'NONE', #15132 ) ;
#11981=ORIENTED_EDGE ( 'NONE', *, *, #16011, .T. ) ;
#11988=EDGE_CURVE ( 'NONE', #3590, #17715, #18571, .T. ) ;
#11998=LINE ( 'NONE', #11803, #17291 ) ;
#12028=VERTEX_POINT ( 'NONE', #2092 ) ;
#12031=CARTESIAN_POINT ( 'NONE',  ( 41.99999999999997868, 139.6861997365471950, 51.99999999999997868 ) ) ;
#12043=ORIENTED_EDGE ( 'NONE', *, *, #11767, .F. ) ;
#12051=PLANE ( 'NONE',  #8144 ) ;
#12057=CARTESIAN_POINT ( 'NONE',  ( -1.040834085586084257E-14, 27.62132034355962773, 54.62132034355965260 ) ) ;
#12058=ORIENTED_EDGE ( 'NONE', *, *, #18875, .F. ) ;
#12063=VECTOR ( 'NONE', #18514, 1000.000000000000000 ) ;
#12084=EDGE_CURVE ( 'NONE', #18422, #9008, #6608, .T. ) ;
#12100=CARTESIAN_POINT ( 'NONE',  ( 50.00000000000000000, 118.0000000000000142, -56.99999999999999289 ) ) ;
#12124=CARTESIAN_POINT ( 'NONE',  ( -1.040834085586084257E-14, 27.62132034355962773, 54.62132034355965260 ) ) ;
#12135=EDGE_CURVE ( 'NONE', #15077, #5315, #9625, .T. ) ;
#12161=LINE ( 'NONE', #13336, #14451 ) ;
#12162=AXIS2_PLACEMENT_3D ( 'NONE', #6905, #2585, #2681 ) ;
#12183=CARTESIAN_POINT ( 'NONE',  ( 43.49999999999997868, 115.0000000000000000, -52.50000000000002132 ) ) ;
#12202=CARTESIAN_POINT ( 'NONE',  ( -41.99999999999997868, 3.000000000000000000, 0.000000000000000000 ) ) ;
#12203=DIRECTION ( 'NONE',  ( 0.000000000000000000, -0.000000000000000000, 1.000000000000000000 ) ) ;
#12222=CYLINDRICAL_SURFACE ( 'NONE', #4784, 10.00000000000000000 ) ;
#12225=VERTEX_POINT ( 'NONE', #2558 ) ;
#12239=( GEOMETRIC_REPRESENTATION_CONTEXT ( 3 ) GLOBAL_UNCERTAINTY_ASSIGNED_CONTEXT ( ( #11384 ) ) GLOBAL_UNIT_ASSIGNED_CONTEXT ( ( #403, #6288, #6481 ) ) REPRESENTATION_CONTEXT ( 'NONE', 'WORKASPACE' ) );
#12263=FACE_BOUND ( 'NONE', #13086, .T. ) ;
#12303=FACE_OUTER_BOUND ( 'NONE', #9755, .T. ) ;
#12315=ORIENTED_EDGE ( 'NONE', *, *, #11372, .F. ) ;
#12319=ORIENTED_EDGE ( 'NONE', *, *, #14705, .T. ) ;
#12321=CARTESIAN_POINT ( 'NONE',  ( -41.99999999999997868, 6.000000000000005329, 51.99999999999997868 ) ) ;
#12326=VERTEX_POINT ( 'NONE', #5317 ) ;
#12327=CARTESIAN_POINT ( 'NONE',  ( 49.99999999999998579, 3.000000000000000000, 59.99999999999997868 ) ) ;
#12336=ORIENTED_EDGE ( 'NONE', *, *, #12707, .F. ) ;
#12381=LINE ( 'NONE', #10904, #18006 ) ;
#12383=ADVANCED_FACE ( 'NONE', ( #4527 ), #110, .F. ) ;
#12386=ADVANCED_FACE ( 'NONE', ( #3047 ), #18056, .F. ) ;
#12389=VECTOR ( 'NONE', #16788, 1000.000000000000000 ) ;
#12397=DIRECTION ( 'NONE',  ( -1.000000000000000000, 0.000000000000000000, 8.163404592832032733E-17 ) ) ;
#12424=EDGE_CURVE ( 'NONE', #13301, #4424, #14816, .T. ) ;
#12434=ORIENTED_EDGE ( 'NONE', *, *, #18994, .T. ) ;
#12477=FACE_OUTER_BOUND ( 'NONE', #17933, .T. ) ;
#12513=CARTESIAN_POINT ( 'NONE',  ( -47.00000000000002132, 6.000000000000000000, -57.00000000000001421 ) ) ;
#12522=LINE ( 'NONE', #16751, #16359 ) ;
#12532=ORIENTED_EDGE ( 'NONE', *, *, #4394, .F. ) ;
#12534=LINE ( 'NONE', #16862, #14608 ) ;
#12535=VERTEX_POINT ( 'NONE', #9603 ) ;
#12541=LINE ( 'NONE', #9687, #8208 ) ;
#12543=PLANE ( 'NONE',  #5026 ) ;
#12564=EDGE_CURVE ( 'NONE', #13301, #1710, #15209, .T. ) ;
#12579=CARTESIAN_POINT ( 'NONE',  ( -1.040834085586084257E-14, 27.62132034355962773, 54.62132034355965260 ) ) ;
#12588=AXIS2_PLACEMENT_3D ( 'NONE', #16151, #8693, #1254 ) ;
#12628=VERTEX_POINT ( 'NONE', #13920 ) ;
#12653=VERTEX_POINT ( 'NONE', #10685 ) ;
#12677=AXIS2_PLACEMENT_3D ( 'NONE', #9319, #3249, #1979 ) ;
#12682=CARTESIAN_POINT ( 'NONE',  ( 49.99999999999998579, 17.99999999999993250, 59.99999999999997868 ) ) ;
#12693=ORIENTED_EDGE ( 'NONE', *, *, #5992, .T. ) ;
#12696=APPLICATION_CONTEXT ( 'automotive_design' ) ;
#12699=AXIS2_PLACEMENT_3D ( 'NONE', #17508, #13191, #17610 ) ;
#12704=CARTESIAN_POINT ( 'NONE',  ( 46.99999999999998579, 115.0000000000000000, 59.99999999999997868 ) ) ;
#12707=EDGE_CURVE ( 'NONE', #17051, #8350, #18152, .T. ) ;
#12734=FACE_OUTER_BOUND ( 'NONE', #167, .T. ) ;
#12742=ORIENTED_EDGE ( 'NONE', *, *, #4115, .T. ) ;
#12746=CARTESIAN_POINT ( 'NONE',  ( -1.040834085586084257E-14, 25.49999999999996803, 52.49999999999998579 ) ) ;
#12747=VERTEX_POINT ( 'NONE', #10878 ) ;
#12753=EDGE_LOOP ( 'NONE', ( #8723, #200, #8803, #15131, #205 ) ) ;
#12756=CARTESIAN_POINT ( 'NONE',  ( 21.49999999999997513, 115.0000000000000000, -52.50000000000002132 ) ) ;
#12764=EDGE_CURVE ( 'NONE', #9008, #14646, #17535, .T. ) ;
#12797=CARTESIAN_POINT ( 'NONE',  ( -1.040834085586084257E-14, 19.13603896932104220, 54.62132034355960286 ) ) ;
#12813=AXIS2_PLACEMENT_3D ( 'NONE', #14387, #16056, #963 ) ;
#12814=CARTESIAN_POINT ( 'NONE',  ( -50.00000000000001421, 118.0000000000000142, 59.99999999999997868 ) ) ;
#12837=ORIENTED_EDGE ( 'NONE', *, *, #13937, .F. ) ;
#12848=PLANE ( 'NONE',  #2804 ) ;
#12856=CARTESIAN_POINT ( 'NONE',  ( -1.040834085586084257E-14, 34.69238815542512100, 47.55025253169419841 ) ) ;
#12876=EDGE_CURVE ( 'NONE', #3207, #4412, #6848, .T. ) ;
#12884=ORIENTED_EDGE ( 'NONE', *, *, #665, .F. ) ;
#12891=ORIENTED_EDGE ( 'NONE', *, *, #9348, .F. ) ;
#12893=DIRECTION ( 'NONE',  ( 0.000000000000000000, 0.7071067811865456854, 0.7071067811865494601 ) ) ;
#12894=EDGE_CURVE ( 'NONE', #12535, #12747, #5291, .T. ) ;
#12937=ORIENTED_EDGE ( 'NONE', *, *, #17165, .F. ) ;
#12971=LINE ( 'NONE', #5735, #7080 ) ;
#12990=EDGE_LOOP ( 'NONE', ( #2717, #7356, #4413, #18545, #18047, #4909, #3262, #743 ) ) ;
#12998=ADVANCED_FACE ( 'NONE', ( #4477 ), #7500, .F. ) ;
#13001=DIRECTION ( 'NONE',  ( -0.000000000000000000, -1.000000000000000000, -0.000000000000000000 ) ) ;
#13011=PLANE ( 'NONE',  #2778 ) ;
#13018=DIRECTION ( 'NONE',  ( 1.000000000000000000, 0.000000000000000000, 0.000000000000000000 ) ) ;
#13019=ORIENTED_EDGE ( 'NONE', *, *, #13961, .F. ) ;
#13024=ORIENTED_EDGE ( 'NONE', *, *, #8836, .F. ) ;
#13029=ORIENTED_EDGE ( 'NONE', *, *, #5881, .F. ) ;
#13036=DIRECTION ( 'NONE',  ( -0.000000000000000000, -0.7071067811865456854, -0.7071067811865493491 ) ) ;
#13037=CARTESIAN_POINT ( 'NONE',  ( -9.183694056713489507E-15, 18.42893218813449607, 59.57106781186546129 ) ) ;
#13043=VERTEX_POINT ( 'NONE', #19367 ) ;
#13047=ADVANCED_FACE ( 'NONE', ( #12303 ), #152, .F. ) ;
#13048=ADVANCED_FACE ( 'NONE', ( #15153 ), #6138, .T. ) ;
#13051=ORIENTED_EDGE ( 'NONE', *, *, #12135, .F. ) ;
#13085=CARTESIAN_POINT ( 'NONE',  ( -21.50000000000000000, 2.999000000000001442, -52.50000000000000711 ) ) ;
#13086=EDGE_LOOP ( 'NONE', ( #1073, #18654 ) ) ;
#13116=ORIENTED_EDGE ( 'NONE', *, *, #8690, .F. ) ;
#13133=CARTESIAN_POINT ( 'NONE',  ( -21.50000000000000000, 115.0000000000000000, 32.50000000000000000 ) ) ;
#13154=EDGE_LOOP ( 'NONE', ( #265, #6263, #10963, #15455 ) ) ;
#13155=AXIS2_PLACEMENT_3D ( 'NONE', #9413, #13831, #112 ) ;
#13167=DIRECTION ( 'NONE',  ( 0.000000000000000000, 0.000000000000000000, -1.000000000000000000 ) ) ;
#13191=DIRECTION ( 'NONE',  ( 0.000000000000000000, -0.7071067811865455743, -0.7071067811865495711 ) ) ;
#13193=ORIENTED_EDGE ( 'NONE', *, *, #6762, .F. ) ;
#13204=ORIENTED_EDGE ( 'NONE', *, *, #13553, .F. ) ;
#13217=CARTESIAN_POINT ( 'NONE',  ( 2.750000000000009770, 38.00000000000000000, -42.68883962248118991 ) ) ;
#13222=CARTESIAN_POINT ( 'NONE',  ( 44.99999999999998579, 3.000000000000000000, -53.49999999999998579 ) ) ;
#13301=VERTEX_POINT ( 'NONE', #12682 ) ;
#13302=CARTESIAN_POINT ( 'NONE',  ( -2.750000000000019540, 115.0000000000000000, 37.49999999999997158 ) ) ;
#13316=ADVANCED_FACE ( 'NONE', ( #9744 ), #15736, .F. ) ;
#13333=CARTESIAN_POINT ( 'NONE',  ( -50.00000000000002132, 33.00000000000000000, 59.99999999999997868 ) ) ;
#13336=CARTESIAN_POINT ( 'NONE',  ( 43.50000000000001421, 2.999000000000001442, 32.49999999999998579 ) ) ;
#13340=VECTOR ( 'NONE', #11361, 1000.000000000000000 ) ;
#13353=ORIENTED_EDGE ( 'NONE', *, *, #4629, .F. ) ;
#13357=DIRECTION ( 'NONE',  ( -0.000000000000000000, -1.000000000000000000, -0.000000000000000000 ) ) ;
#13366=DIRECTION ( 'NONE',  ( -1.000000000000000000, 0.000000000000000000, -1.156482317317871725E-16 ) ) ;
#13378=DIRECTION ( 'NONE',  ( 0.000000000000000000, 0.000000000000000000, -1.000000000000000000 ) ) ;
#13385=VERTEX_POINT ( 'NONE', #19052 ) ;
#13400=EDGE_LOOP ( 'NONE', ( #2270, #6648 ) ) ;
#13405=DIRECTION ( 'NONE',  ( 0.000000000000000000, 0.000000000000000000, -1.000000000000000000 ) ) ;
#13413=ORIENTED_EDGE ( 'NONE', *, *, #6863, .T. ) ;
#13416=EDGE_CURVE ( 'NONE', #7552, #10804, #1019, .T. ) ;
#13439=VERTEX_POINT ( 'NONE', #17585 ) ;
#13456=EDGE_CURVE ( 'NONE', #4041, #7547, #5164, .T. ) ;
#13506=AXIS2_PLACEMENT_3D ( 'NONE', #3247, #2160, #11073 ) ;
#13551=ORIENTED_EDGE ( 'NONE', *, *, #12564, .T. ) ;
#13553=EDGE_CURVE ( 'NONE', #2359, #10684, #1512, .T. ) ;
#13567=EDGE_CURVE ( 'NONE', #18422, #1873, #9535, .T. ) ;
#13571=CARTESIAN_POINT ( 'NONE',  ( 43.50000000000001421, 2.999000000000001442, 32.49999999999998579 ) ) ;
#13574=FACE_OUTER_BOUND ( 'NONE', #15421, .T. ) ;
#13581=VECTOR ( 'NONE', #16286, 1000.000000000000000 ) ;
#13593=CARTESIAN_POINT ( 'NONE',  ( -2.749999999999988454, 37.99999999999999289, 40.49999999999996447 ) ) ;
#13599=CARTESIAN_POINT ( 'NONE',  ( 41.99999999999997868, 6.000000000000005329, 51.99999999999997868 ) ) ;
#13600=LINE ( 'NONE', #8896, #10039 ) ;
#13629=CIRCLE ( 'NONE', #14560, 6.000000000000003553 ) ;
#13642=AXIS2_PLACEMENT_3D ( 'NONE', #18673, #9538, #5143 ) ;
#13660=EDGE_CURVE ( 'NONE', #16697, #11555, #2965, .T. ) ;
#13670=DIRECTION ( 'NONE',  ( -2.081668171172167774E-16, 0.000000000000000000, 1.000000000000000000 ) ) ;
#13676=DIRECTION ( 'NONE',  ( -0.000000000000000000, 1.000000000000000000, 1.632680918566406547E-16 ) ) ;
#13684=ORIENTED_EDGE ( 'NONE', *, *, #10439, .T. ) ;
#13713=CARTESIAN_POINT ( 'NONE',  ( 0.000000000000000000, 0.000000000000000000, 0.000000000000000000 ) ) ;
#13715=ORIENTED_EDGE ( 'NONE', *, *, #3155, .T. ) ;
#13722=SURFACE_SIDE_STYLE ('',( #16975 ) ) ;
#13732=DIRECTION ( 'NONE',  ( -0.000000000000000000, 1.000000000000000000, -0.000000000000000000 ) ) ;
#13733=VECTOR ( 'NONE', #16334, 1000.000000000000000 ) ;
#13736=CARTESIAN_POINT ( 'NONE',  ( -43.50000000000000711, 118.0000000000000142, -52.50000000000000711 ) ) ;
#13739=CARTESIAN_POINT ( 'NONE',  ( -41.99999999999997868, 6.000000000000005329, -52.00000000000000000 ) ) ;
#13774=DIRECTION ( 'NONE',  ( 0.000000000000000000, 0.000000000000000000, -1.000000000000000000 ) ) ;
#13775=DIRECTION ( 'NONE',  ( -0.000000000000000000, -1.000000000000000000, -0.000000000000000000 ) ) ;
#13792=VECTOR ( 'NONE', #3819, 1000.000000000000114 ) ;
#13795=EDGE_LOOP ( 'NONE', ( #482, #14381, #6724, #19346 ) ) ;
#13797=PLANE ( 'NONE',  #4428 ) ;
#13806=FACE_OUTER_BOUND ( 'NONE', #13795, .T. ) ;
#13823=ORIENTED_EDGE ( 'NONE', *, *, #11284, .T. ) ;
#13824=ADVANCED_FACE ( 'NONE', ( #11003 ), #9533, .F. ) ;
#13827=EDGE_LOOP ( 'NONE', ( #3068, #16968, #18624, #11340, #3364, #7584, #4288 ) ) ;
#13831=DIRECTION ( 'NONE',  ( 0.000000000000000000, 1.000000000000000000, 0.000000000000000000 ) ) ;
#13835=AXIS2_PLACEMENT_3D ( 'NONE', #15063, #2901, #4184 ) ;
#13856=CARTESIAN_POINT ( 'NONE',  ( -44.99999999999998579, 3.000000000000000000, -53.50000000000000000 ) ) ;
#13873=DIRECTION ( 'NONE',  ( 1.000000000000000000, -0.000000000000000000, 0.000000000000000000 ) ) ;
#13874=FACE_BOUND ( 'NONE', #13400, .T. ) ;
#13896=CARTESIAN_POINT ( 'NONE',  ( 2.749999999999979128, 118.0000000000000142, 37.49999999999997158 ) ) ;
#13899=VECTOR ( 'NONE', #16019, 1000.000000000000000 ) ;
#13904=ORIENTED_EDGE ( 'NONE', *, *, #7448, .T. ) ;
#13907=ORIENTED_EDGE ( 'NONE', *, *, #2678, .T. ) ;
#13910=EDGE_CURVE ( 'NONE', #7059, #13385, #12381, .T. ) ;
#13920=CARTESIAN_POINT ( 'NONE',  ( -50.00000000000002132, 33.00000000000000000, 40.49999999999996447 ) ) ;
#13921=ORIENTED_EDGE ( 'NONE', *, *, #744, .F. ) ;
#13937=EDGE_CURVE ( 'NONE', #5315, #587, #6974, .T. ) ;
#13939=FACE_OUTER_BOUND ( 'NONE', #11186, .T. ) ;
#13961=EDGE_CURVE ( 'NONE', #12028, #19093, #18937, .T. ) ;
#13972=AXIS2_PLACEMENT_3D ( 'NONE', #16119, #13366, #4266 ) ;
#14000=CARTESIAN_POINT ( 'NONE',  ( -21.50000000000000000, 118.0000000000000142, 32.50000000000000000 ) ) ;
#14040=ORIENTED_EDGE ( 'NONE', *, *, #5328, .F. ) ;
#14054=VERTEX_POINT ( 'NONE', #898 ) ;
#14055=CIRCLE ( 'NONE', #2167, 6.000000000000003553 ) ;
#14060=EDGE_CURVE ( 'NONE', #17940, #18716, #5418, .T. ) ;
#14093=AXIS2_PLACEMENT_3D ( 'NONE', #18283, #4852, #9338 ) ;
#14096=CARTESIAN_POINT ( 'NONE',  ( -9.551088096457694952E-15, 22.67157287525377996, 59.57106781186547551 ) ) ;
#14100=DIRECTION ( 'NONE',  ( 1.000000000000000000, 0.000000000000000000, 0.000000000000000000 ) ) ;
#14126=MECHANICAL_DESIGN_GEOMETRIC_PRESENTATION_REPRESENTATION('',(#5977),#12239);
#14155=ORIENTED_EDGE ( 'NONE', *, *, #2081, .T. ) ;
#14182=CARTESIAN_POINT ( 'NONE',  ( 43.50000000000001421, 115.0000000000000000, 32.49999999999998579 ) ) ;
#14200=EDGE_LOOP ( 'NONE', ( #8617, #8028 ) ) ;
#14205=LINE ( 'NONE', #11154, #14767 ) ;
#14238=DIRECTION ( 'NONE',  ( -0.000000000000000000, -1.000000000000000000, -0.000000000000000000 ) ) ;
#14244=ORIENTED_EDGE ( 'NONE', *, *, #17493, .T. ) ;
#14245=DIRECTION ( 'NONE',  ( 0.000000000000000000, 0.7071067811865492381, -0.7071067811865456854 ) ) ;
#14265=ORIENTED_EDGE ( 'NONE', *, *, #3776, .T. ) ;
#14266=ADVANCED_FACE ( 'NONE', ( #1684 ), #214, .F. ) ;
#14279=LINE ( 'NONE', #15940, #11211 ) ;
#14285=ORIENTED_EDGE ( 'NONE', *, *, #11868, .T. ) ;
#14301=ADVANCED_FACE ( 'NONE', ( #9417 ), #18354, .F. ) ;
#14310=ADVANCED_FACE ( 'NONE', ( #16686 ), #3443, .F. ) ;
#14314=ORIENTED_EDGE ( 'NONE', *, *, #11267, .T. ) ;
#14316=FACE_OUTER_BOUND ( 'NONE', #7981, .T. ) ;
#14320=EDGE_CURVE ( 'NONE', #11555, #16697, #15506, .T. ) ;
#14334=ORIENTED_EDGE ( 'NONE', *, *, #8229, .F. ) ;
#14364=AXIS2_PLACEMENT_3D ( 'NONE', #18553, #8249, #9511 ) ;
#14381=ORIENTED_EDGE ( 'NONE', *, *, #2678, .F. ) ;
#14384=VECTOR ( 'NONE', #5285, 1000.000000000000114 ) ;
#14385=FACE_OUTER_BOUND ( 'NONE', #11727, .T. ) ;
#14387=CARTESIAN_POINT ( 'NONE',  ( -44.99999999999998579, 3.000000000000000000, -55.00000000000000000 ) ) ;
#14403=DIRECTION ( 'NONE',  ( 0.000000000000000000, 1.000000000000000000, 1.632680918566406793E-16 ) ) ;
#14418=ORIENTED_EDGE ( 'NONE', *, *, #16188, .T. ) ;
#14436=VECTOR ( 'NONE', #8544, 1000.000000000000000 ) ;
#14451=VECTOR ( 'NONE', #13732, 1000.000000000000000 ) ;
#14479=ORIENTED_EDGE ( 'NONE', *, *, #16094, .T. ) ;
#14487=LINE ( 'NONE', #2255, #3164 ) ;
#14488=ORIENTED_EDGE ( 'NONE', *, *, #16748, .F. ) ;
#14526=ORIENTED_EDGE ( 'NONE', *, *, #13553, .T. ) ;
#14536=CARTESIAN_POINT ( 'NONE',  ( 21.50000000000001421, 118.0000000000000142, 32.49999999999998579 ) ) ;
#14543=EDGE_CURVE ( 'NONE', #13439, #3909, #16784, .T. ) ;
#14545=CARTESIAN_POINT ( 'NONE',  ( -50.00000000000002132, 118.0000000000000142, 40.49999999999997868 ) ) ;
#14552=VERTEX_POINT ( 'NONE', #12513 ) ;
#14560=AXIS2_PLACEMENT_3D ( 'NONE', #6302, #1689, #16885 ) ;
#14568=DIRECTION ( 'NONE',  ( -1.000000000000000000, 0.000000000000000000, -2.081668171172167774E-16 ) ) ;
#14571=VERTEX_POINT ( 'NONE', #12321 ) ;
#14605=LINE ( 'NONE', #19023, #8053 ) ;
#14608=VECTOR ( 'NONE', #16671, 1000.000000000000000 ) ;
#14611=ORIENTED_EDGE ( 'NONE', *, *, #2292, .F. ) ;
#14617=DIRECTION ( 'NONE',  ( 5.782411586589357392E-17, 0.000000000000000000, 1.000000000000000000 ) ) ;
#14643=DIRECTION ( 'NONE',  ( 0.000000000000000000, -1.000000000000000000, 0.000000000000000000 ) ) ;
#14646=VERTEX_POINT ( 'NONE', #5262 ) ;
#14649=EDGE_CURVE ( 'NONE', #12225, #4598, #2223, .T. ) ;
#14660=AXIS2_PLACEMENT_3D ( 'NONE', #2602, #9854, #4079 ) ;
#14679=ORIENTED_EDGE ( 'NONE', *, *, #10487, .F. ) ;
#14682=ORIENTED_EDGE ( 'NONE', *, *, #13937, .T. ) ;
#14683=ORIENTED_EDGE ( 'NONE', *, *, #14649, .F. ) ;
#14687=VECTOR ( 'NONE', #18659, 1000.000000000000000 ) ;
#14689=DIRECTION ( 'NONE',  ( -0.000000000000000000, -0.000000000000000000, 1.000000000000000000 ) ) ;
#14705=EDGE_CURVE ( 'NONE', #7257, #13043, #3594, .T. ) ;
#14721=CARTESIAN_POINT ( 'NONE',  ( -50.00000000000002132, 118.0000000000000142, -60.00000000000002132 ) ) ;
#14737=DIRECTION ( 'NONE',  ( -1.000000000000000000, 0.000000000000000000, 0.000000000000000000 ) ) ;
#14745=PRODUCT_DEFINITION_SHAPE ( 'NONE', 'NONE',  #4165 ) ;
#14753=VECTOR ( 'NONE', #2623, 1000.000000000000000 ) ;
#14765=LINE ( 'NONE', #6046, #6234 ) ;
#14767=VECTOR ( 'NONE', #11062, 1000.000000000000000 ) ;
#14785=AXIS2_PLACEMENT_3D ( 'NONE', #15539, #2110, #7797 ) ;
#14788=ORIENTED_EDGE ( 'NONE', *, *, #11868, .F. ) ;
#14789=ORIENTED_EDGE ( 'NONE', *, *, #18004, .F. ) ;
#14793=FACE_BOUND ( 'NONE', #11521, .T. ) ;
#14795=CARTESIAN_POINT ( 'NONE',  ( 43.50000000000001421, 2.999000000000001442, 32.49999999999998579 ) ) ;
#14800=CARTESIAN_POINT ( 'NONE',  ( 43.49999999999997868, 118.0000000000000142, -52.50000000000002132 ) ) ;
#14810=DIRECTION ( 'NONE',  ( 1.000000000000000000, 0.000000000000000000, 0.000000000000000000 ) ) ;
#14812=ORIENTED_EDGE ( 'NONE', *, *, #757, .T. ) ;
#14816=LINE ( 'NONE', #4630, #10627 ) ;
#14846=DIRECTION ( 'NONE',  ( 1.000000000000000000, 0.000000000000000000, 0.000000000000000000 ) ) ;
#14859=LINE ( 'NONE', #11809, #11828 ) ;
#14886=DIRECTION ( 'NONE',  ( -1.000000000000000000, 0.000000000000000000, -0.000000000000000000 ) ) ;
#14908=ORIENTED_EDGE ( 'NONE', *, *, #3846, .T. ) ;
#14918=LINE ( 'NONE', #1490, #6612 ) ;
#14942=DIRECTION ( 'NONE',  ( -0.000000000000000000, 1.000000000000000000, -0.000000000000000000 ) ) ;
#14996=EDGE_LOOP ( 'NONE', ( #16863, #12891 ) ) ;
#15001=LINE ( 'NONE', #2842, #19084 ) ;
#15033=EDGE_LOOP ( 'NONE', ( #9333, #17248, #16250, #18815 ) ) ;
#15046=EDGE_CURVE ( 'NONE', #587, #18462, #551, .T. ) ;
#15058=DIRECTION ( 'NONE',  ( 1.000000000000000000, 0.000000000000000000, 0.000000000000000000 ) ) ;
#15063=CARTESIAN_POINT ( 'NONE',  ( 44.99999999999998579, 6.000000000000000000, -54.99999999999998579 ) ) ;
#15068=VECTOR ( 'NONE', #2001, 1000.000000000000000 ) ;
#15077=VERTEX_POINT ( 'NONE', #11400 ) ;
#15084=VERTEX_POINT ( 'NONE', #9753 ) ;
#15085=ORIENTED_EDGE ( 'NONE', *, *, #2297, .T. ) ;
#15097=VERTEX_POINT ( 'NONE', #5445 ) ;
#15098=ORIENTED_EDGE ( 'NONE', *, *, #11028, .T. ) ;
#15100=AXIS2_PLACEMENT_3D ( 'NONE', #10829, #6142, #12203 ) ;
#15109=LINE ( 'NONE', #9122, #15995 ) ;
#15131=ORIENTED_EDGE ( 'NONE', *, *, #13910, .F. ) ;
#15132=CARTESIAN_POINT ( 'NONE',  ( 21.50000000000001421, 118.0000000000000142, 32.49999999999998579 ) ) ;
#15134=DIRECTION ( 'NONE',  ( 3.826732013112563602E-16, -1.000000000000000000, 0.000000000000000000 ) ) ;
#15141=CARTESIAN_POINT ( 'NONE',  ( 41.99999999999998579, 6.000000000000005329, -52.00000000000000000 ) ) ;
#15153=FACE_OUTER_BOUND ( 'NONE', #7297, .T. ) ;
#15156=FACE_BOUND ( 'NONE', #15267, .T. ) ;
#15170=( LENGTH_UNIT ( ) NAMED_UNIT ( * ) SI_UNIT ( .MILLI., .METRE. ) );
#15180=EDGE_LOOP ( 'NONE', ( #3432, #18446, #3892, #2258 ) ) ;
#15183=ORIENTED_EDGE ( 'NONE', *, *, #19206, .T. ) ;
#15195=PRODUCT_DEFINITION_FORMATION_WITH_SPECIFIED_SOURCE ( 'ANY', '', #5998, .NOT_KNOWN. ) ;
#15197=ORIENTED_EDGE ( 'NONE', *, *, #10385, .T. ) ;
#15207=CARTESIAN_POINT ( 'NONE',  ( -1.040834085586084257E-14, 32.57106781186548972, 45.42893218813454581 ) ) ;
#15209=LINE ( 'NONE', #495, #18495 ) ;
#15212=FACE_BOUND ( 'NONE', #14200, .T. ) ;
#15234=CARTESIAN_POINT ( 'NONE',  ( -2.750000000000020872, 118.0000000000000142, -42.68883962248118991 ) ) ;
#15255=PLANE ( 'NONE',  #10905 ) ;
#15263=ORIENTED_EDGE ( 'NONE', *, *, #4104, .T. ) ;
#15267=EDGE_LOOP ( 'NONE', ( #3246, #16647 ) ) ;
#15284=ORIENTED_EDGE ( 'NONE', *, *, #18144, .T. ) ;
#15297=EDGE_LOOP ( 'NONE', ( #12742, #4202, #4132, #16303 ) ) ;
#15309=VECTOR ( 'NONE', #2990, 1000.000000000000000 ) ;
#15312=VERTEX_POINT ( 'NONE', #4170 ) ;
#15321=ORIENTED_EDGE ( 'NONE', *, *, #11988, .T. ) ;
#15324=FACE_OUTER_BOUND ( 'NONE', #174, .T. ) ;
#15341=VECTOR ( 'NONE', #5267, 1000.000000000000000 ) ;
#15350=CARTESIAN_POINT ( 'NONE',  ( -41.99999999999997868, 139.6861997365471950, 51.99999999999997868 ) ) ;
#15355=ADVANCED_FACE ( 'NONE', ( #10417 ), #1121, .F. ) ;
#15360=ORIENTED_EDGE ( 'NONE', *, *, #17296, .F. ) ;
#15364=( NAMED_UNIT ( * ) SI_UNIT ( $, .STERADIAN. ) SOLID_ANGLE_UNIT ( ) );
#15385=AXIS2_PLACEMENT_3D ( 'NONE', #1459, #10155, #14886 ) ;
#15388=EDGE_CURVE ( 'NONE', #12747, #17810, #12971, .T. ) ;
#15407=FACE_OUTER_BOUND ( 'NONE', #1441, .T. ) ;
#15409=CARTESIAN_POINT ( 'NONE',  ( -21.50000000000000000, 2.999000000000001442, 32.50000000000000000 ) ) ;
#15421=EDGE_LOOP ( 'NONE', ( #12937, #18442, #16032, #7147 ) ) ;
#15432=DIRECTION ( 'NONE',  ( 0.000000000000000000, -0.000000000000000000, 1.000000000000000000 ) ) ;
#15455=ORIENTED_EDGE ( 'NONE', *, *, #16839, .F. ) ;
#15459=ORIENTED_EDGE ( 'NONE', *, *, #12894, .F. ) ;
#15483=ORIENTED_EDGE ( 'NONE', *, *, #11511, .F. ) ;
#15487=( GEOMETRIC_REPRESENTATION_CONTEXT ( 3 ) GLOBAL_UNCERTAINTY_ASSIGNED_CONTEXT ( ( #1794 ) ) GLOBAL_UNIT_ASSIGNED_CONTEXT ( ( #15170, #7722, #15364 ) ) REPRESENTATION_CONTEXT ( 'NONE', 'WORKASPACE' ) );
#15495=DIRECTION ( 'NONE',  ( 1.156482317317871725E-16, 0.000000000000000000, -1.000000000000000000 ) ) ;
#15506=CIRCLE ( 'NONE', #12677, 1.500000000000001332 ) ;
#15539=CARTESIAN_POINT ( 'NONE',  ( -44.99999999999998579, 6.000000000000000000, -55.00000000000000000 ) ) ;
#15557=VECTOR ( 'NONE', #9421, 1000.000000000000000 ) ;
#15576=EDGE_LOOP ( 'NONE', ( #9772, #12532, #13353, #18562 ) ) ;
#15579=ORIENTED_EDGE ( 'NONE', *, *, #6499, .T. ) ;
#15604=DIRECTION ( 'NONE',  ( 0.000000000000000000, -0.7071067811865455743, -0.7071067811865495711 ) ) ;
#15610=CARTESIAN_POINT ( 'NONE',  ( -50.00000000000002132, 115.0000000000000000, 37.49999999999997868 ) ) ;
#15611=ORIENTED_EDGE ( 'NONE', *, *, #9348, .T. ) ;
#15613=DIRECTION ( 'NONE',  ( -0.000000000000000000, -0.7071067811865456854, -0.7071067811865494601 ) ) ;
#15619=PLANE ( 'NONE',  #7235 ) ;
#15659=CARTESIAN_POINT ( 'NONE',  ( 21.50000000000001421, 115.0000000000000000, 32.49999999999998579 ) ) ;
#15667=VECTOR ( 'NONE', #14689, 1000.000000000000000 ) ;
#15673=ORIENTED_EDGE ( 'NONE', *, *, #3882, .F. ) ;
#15680=DIRECTION ( 'NONE',  ( 1.000000000000000000, 0.000000000000000000, 0.000000000000000000 ) ) ;
#15686=LINE ( 'NONE', #5390, #13792 ) ;
#15700=ORIENTED_EDGE ( 'NONE', *, *, #15388, .T. ) ;
#15715=CARTESIAN_POINT ( 'NONE',  ( -9.551088096457694952E-15, 20.55025253169411670, 57.44974746830580870 ) ) ;
#15719=VECTOR ( 'NONE', #5568, 1000.000000000000000 ) ;
#15726=ADVANCED_FACE ( 'NONE', ( #6798, #18756, #11103 ), #2002, .T. ) ;
#15736=PLANE ( 'NONE',  #17368 ) ;
#15741=CYLINDRICAL_SURFACE ( 'NONE', #12162, 1.500000000000001332 ) ;
#15779=ORIENTED_EDGE ( 'NONE', *, *, #16839, .T. ) ;
#15784=DIRECTION ( 'NONE',  ( 0.000000000000000000, -0.7071067811865493491, 0.7071067811865456854 ) ) ;
#15797=VECTOR ( 'NONE', #15809, 1000.000000000000114 ) ;
#15799=LINE ( 'NONE', #2552, #3122 ) ;
#15805=LINE ( 'NONE', #5233, #16270 ) ;
#15807=LINE ( 'NONE', #8543, #32 ) ;
#15809=DIRECTION ( 'NONE',  ( -0.000000000000000000, -0.7071067811865456854, -0.7071067811865493491 ) ) ;
#15829=CIRCLE ( 'NONE', #3931, 10.00000000000000178 ) ;
#15832=DIRECTION ( 'NONE',  ( -0.000000000000000000, -1.000000000000000000, -0.000000000000000000 ) ) ;
#15871=DIRECTION ( 'NONE',  ( -6.672013369141567928E-17, 0.000000000000000000, 1.000000000000000000 ) ) ;
#15882=DIRECTION ( 'NONE',  ( 0.000000000000000000, 1.632680918566406793E-16, -1.000000000000000000 ) ) ;
#15883=EDGE_LOOP ( 'NONE', ( #7644, #7173, #6789, #5000 ) ) ;
#15889=CARTESIAN_POINT ( 'NONE',  ( -44.99999999999998579, 3.000000000000000000, -56.50000000000000000 ) ) ;
#15897=DIRECTION ( 'NONE',  ( 1.156482317317871725E-16, 0.000000000000000000, -1.000000000000000000 ) ) ;
#15935=VERTEX_POINT ( 'NONE', #4337 ) ;
#15938=VECTOR ( 'NONE', #17164, 1000.000000000000000 ) ;
#15940=CARTESIAN_POINT ( 'NONE',  ( 46.99999999999997868, 30.87867965644035806, 42.87867965644034740 ) ) ;
#15946=VECTOR ( 'NONE', #1481, 1000.000000000000000 ) ;
#15971=FACE_OUTER_BOUND ( 'NONE', #11883, .T. ) ;
#15995=VECTOR ( 'NONE', #1679, 1000.000000000000000 ) ;
#15998=FACE_OUTER_BOUND ( 'NONE', #3224, .T. ) ;
#16002=VECTOR ( 'NONE', #672, 1000.000000000000114 ) ;
#16011=EDGE_CURVE ( 'NONE', #18238, #11126, #4921, .T. ) ;
#16013=VECTOR ( 'NONE', #13676, 1000.000000000000000 ) ;
#16019=DIRECTION ( 'NONE',  ( 4.898042755699219393E-16, -0.000000000000000000, 1.000000000000000000 ) ) ;
#16032=ORIENTED_EDGE ( 'NONE', *, *, #6499, .F. ) ;
#16054=CARTESIAN_POINT ( 'NONE',  ( 41.99999999999997868, 139.6861997365471950, 51.99999999999997868 ) ) ;
#16056=DIRECTION ( 'NONE',  ( -0.000000000000000000, -1.000000000000000000, -0.000000000000000000 ) ) ;
#16067=LINE ( 'NONE', #11735, #15667 ) ;
#16071=ORIENTED_EDGE ( 'NONE', *, *, #12084, .T. ) ;
#16081=CARTESIAN_POINT ( 'NONE',  ( -50.00000000000001421, 3.000000000000000000, 59.99999999999997868 ) ) ;
#16094=EDGE_CURVE ( 'NONE', #11949, #3590, #6592, .T. ) ;
#16119=CARTESIAN_POINT ( 'NONE',  ( 49.99999999999998579, 118.0000000000000142, 59.99999999999997868 ) ) ;
#16124=CARTESIAN_POINT ( 'NONE',  ( -41.99999999999997868, 3.000000000000002665, 51.99999999999997868 ) ) ;
#16147=ORIENTED_EDGE ( 'NONE', *, *, #16188, .F. ) ;
#16151=CARTESIAN_POINT ( 'NONE',  ( -2.750000000000020872, 118.0000000000000142, -42.68883962248118991 ) ) ;
#16153=CARTESIAN_POINT ( 'NONE',  ( -47.00000000000001421, 16.75735931288065572, 56.99999999999997158 ) ) ;
#16166=DIRECTION ( 'NONE',  ( -0.000000000000000000, -1.000000000000000000, -0.000000000000000000 ) ) ;
#16171=DIRECTION ( 'NONE',  ( -0.000000000000000000, -1.000000000000000000, -0.000000000000000000 ) ) ;
#16188=EDGE_CURVE ( 'NONE', #1873, #14646, #5128, .T. ) ;
#16232=CARTESIAN_POINT ( 'NONE',  ( 46.99999999999998579, 30.00000000000000355, 43.75735931288070191 ) ) ;
#16234=ORIENTED_EDGE ( 'NONE', *, *, #16680, .T. ) ;
#16250=ORIENTED_EDGE ( 'NONE', *, *, #7567, .T. ) ;
#16260=DIRECTION ( 'NONE',  ( 0.000000000000000000, 1.000000000000000000, 0.000000000000000000 ) ) ;
#16263=ORIENTED_EDGE ( 'NONE', *, *, #12876, .T. ) ;
#16265=LINE ( 'NONE', #13222, #7413 ) ;
#16270=VECTOR ( 'NONE', #15897, 1000.000000000000000 ) ;
#16271=CARTESIAN_POINT ( 'NONE',  ( 44.99999999999997158, 6.000000000000000000, 56.50000000000000000 ) ) ;
#16276=CARTESIAN_POINT ( 'NONE',  ( 50.00000000000000000, 118.0000000000000142, -60.00000000000000000 ) ) ;
#16286=DIRECTION ( 'NONE',  ( -1.000000000000000000, 0.000000000000000000, 0.000000000000000000 ) ) ;
#16303=ORIENTED_EDGE ( 'NONE', *, *, #14649, .T. ) ;
#16316=DIRECTION ( 'NONE',  ( -0.000000000000000000, 1.000000000000000000, -0.000000000000000000 ) ) ;
#16321=VECTOR ( 'NONE', #16875, 1000.000000000000000 ) ;
#16331=CARTESIAN_POINT ( 'NONE',  ( -43.50000000000000000, 118.0000000000000142, 32.50000000000000000 ) ) ;
#16334=DIRECTION ( 'NONE',  ( -0.000000000000000000, -0.000000000000000000, 1.000000000000000000 ) ) ;
#16341=CARTESIAN_POINT ( 'NONE',  ( -9.183694056713489507E-15, 20.55025253169413091, 61.69238815542511389 ) ) ;
#16343=ORIENTED_EDGE ( 'NONE', *, *, #1109, .T. ) ;
#16352=AXIS2_PLACEMENT_3D ( 'NONE', #16447, #2917, #1551 ) ;
#16359=VECTOR ( 'NONE', #11138, 1000.000000000000000 ) ;
#16360=ORIENTED_EDGE ( 'NONE', *, *, #3628, .F. ) ;
#16447=CARTESIAN_POINT ( 'NONE',  ( -45.00000000000000000, 3.000000000000000000, 54.99999999999998579 ) ) ;
#16465=ORIENTED_EDGE ( 'NONE', *, *, #11988, .F. ) ;
#16468=CARTESIAN_POINT ( 'NONE',  ( 46.99999999999998579, 118.0000000000000142, 59.99999999999997868 ) ) ;
#16474=EDGE_LOOP ( 'NONE', ( #6352, #8842, #11136, #1650 ) ) ;
#16515=EDGE_LOOP ( 'NONE', ( #3922, #17880, #1668, #19021 ) ) ;
#16523=DIRECTION ( 'NONE',  ( -0.000000000000000000, -1.000000000000000000, -0.000000000000000000 ) ) ;
#16533=ORIENTED_EDGE ( 'NONE', *, *, #11767, .T. ) ;
#16546=EDGE_LOOP ( 'NONE', ( #3500, #6082, #14244, #4419 ) ) ;
#16563=ORIENTED_EDGE ( 'NONE', *, *, #11372, .T. ) ;
#16568=ORIENTED_EDGE ( 'NONE', *, *, #17296, .T. ) ;
#16581=LINE ( 'NONE', #10777, #9099 ) ;
#16593=ORIENTED_EDGE ( 'NONE', *, *, #7567, .F. ) ;
#16647=ORIENTED_EDGE ( 'NONE', *, *, #13456, .F. ) ;
#16655=ORIENTED_EDGE ( 'NONE', *, *, #9621, .T. ) ;
#16659=EDGE_LOOP ( 'NONE', ( #16747, #13715, #1974, #15579, #11423, #5660, #3694 ) ) ;
#16671=DIRECTION ( 'NONE',  ( -1.000000000000000000, 0.000000000000000000, -2.081668171172167774E-16 ) ) ;
#16680=EDGE_CURVE ( 'NONE', #6552, #14552, #831, .T. ) ;
#16686=FACE_OUTER_BOUND ( 'NONE', #13154, .T. ) ;
#16692=LINE ( 'NONE', #7771, #17393 ) ;
#16697=VERTEX_POINT ( 'NONE', #18879 ) ;
#16703=DIRECTION ( 'NONE',  ( -4.081702296416016490E-16, 0.000000000000000000, -1.000000000000000000 ) ) ;
#16711=EDGE_CURVE ( 'NONE', #1741, #5915, #10218, .T. ) ;
#16715=ORIENTED_EDGE ( 'NONE', *, *, #3059, .T. ) ;
#16747=ORIENTED_EDGE ( 'NONE', *, *, #17551, .F. ) ;
#16748=EDGE_CURVE ( 'NONE', #3909, #5783, #17215, .T. ) ;
#16751=CARTESIAN_POINT ( 'NONE',  ( 44.99999999999997158, 3.000000000000000000, 53.50000000000000000 ) ) ;
#16784=CIRCLE ( 'NONE', #3618, 1.500000000000001332 ) ;
#16788=DIRECTION ( 'NONE',  ( -1.000000000000000000, -0.000000000000000000, -0.000000000000000000 ) ) ;
#16801=FACE_BOUND ( 'NONE', #15576, .T. ) ;
#16839=EDGE_CURVE ( 'NONE', #18711, #15312, #10223, .T. ) ;
#16847=ORIENTED_EDGE ( 'NONE', *, *, #10106, .F. ) ;
#16857=ADVANCED_FACE ( 'NONE', ( #12477 ), #3663, .T. ) ;
#16862=CARTESIAN_POINT ( 'NONE',  ( 50.00000000000000000, 115.0000000000000000, -56.99999999999999289 ) ) ;
#16863=ORIENTED_EDGE ( 'NONE', *, *, #18266, .F. ) ;
#16874=VERTEX_POINT ( 'NONE', #18286 ) ;
#16875=DIRECTION ( 'NONE',  ( 1.000000000000000000, 0.000000000000000000, 0.000000000000000000 ) ) ;
#16885=DIRECTION ( 'NONE',  ( 0.000000000000000000, -0.7071067811865492381, 0.7071067811865456854 ) ) ;
#16898=FACE_BOUND ( 'NONE', #6251, .T. ) ;
#16951=CARTESIAN_POINT ( 'NONE',  ( 43.49999999999997868, 118.0000000000000142, -52.50000000000002132 ) ) ;
#16954=CARTESIAN_POINT ( 'NONE',  ( -45.00000000000000000, 6.000000000000000000, 53.49999999999998579 ) ) ;
#16968=ORIENTED_EDGE ( 'NONE', *, *, #6088, .T. ) ;
#16975=SURFACE_STYLE_FILL_AREA ( #4919 ) ;
#16990=CARTESIAN_POINT ( 'NONE',  ( -1.040834085586084257E-14, 27.62132034355962773, 54.62132034355965260 ) ) ;
#16994=FACE_BOUND ( 'NONE', #14996, .T. ) ;
#17003=DIRECTION ( 'NONE',  ( -1.000000000000000000, -3.826732013112563602E-16, 0.000000000000000000 ) ) ;
#17009=LINE ( 'NONE', #4766, #15068 ) ;
#17019=EDGE_CURVE ( 'NONE', #11126, #4048, #9909, .T. ) ;
#17034=FILL_AREA_STYLE_COLOUR ( '', #5163 ) ;
#17041=ORIENTED_EDGE ( 'NONE', *, *, #13416, .T. ) ;
#17044=DIRECTION ( 'NONE',  ( 1.000000000000000000, 0.000000000000000000, 2.081668171172167774E-16 ) ) ;
#17051=VERTEX_POINT ( 'NONE', #2376 ) ;
#17071=LINE ( 'NONE', #3633, #8193 ) ;
#17074=DIRECTION ( 'NONE',  ( 0.000000000000000000, 0.000000000000000000, -1.000000000000000000 ) ) ;
#17118=CARTESIAN_POINT ( 'NONE',  ( 46.99999999999997868, 30.00000000000000355, 59.99999999999999289 ) ) ;
#17150=EDGE_CURVE ( 'NONE', #2227, #869, #3156, .T. ) ;
#17157=ADVANCED_FACE ( 'NONE', ( #1188 ), #1300, .F. ) ;
#17164=DIRECTION ( 'NONE',  ( 0.000000000000000000, 0.000000000000000000, -1.000000000000000000 ) ) ;
#17165=EDGE_CURVE ( 'NONE', #18948, #15097, #19140, .T. ) ;
#17170=CARTESIAN_POINT ( 'NONE',  ( -50.00000000000002132, 118.0000000000000142, 40.49999999999997868 ) ) ;
#17175=CARTESIAN_POINT ( 'NONE',  ( 50.00000000000000000, 33.00000000000000000, 44.99999999999999289 ) ) ;
#17215=LINE ( 'NONE', #5350, #7332 ) ;
#17224=AXIS2_PLACEMENT_3D ( 'NONE', #12057, #10389, #2749 ) ;
#17229=CIRCLE ( 'NONE', #14093, 10.00000000000000178 ) ;
#17230=EDGE_CURVE ( 'NONE', #8073, #18948, #17662, .T. ) ;
#17236=FACE_OUTER_BOUND ( 'NONE', #15297, .T. ) ;
#17242=ORIENTED_EDGE ( 'NONE', *, *, #4130, .F. ) ;
#17248=ORIENTED_EDGE ( 'NONE', *, *, #500, .T. ) ;
#17264=PLANE ( 'NONE',  #10490 ) ;
#17280=DIRECTION ( 'NONE',  ( -5.782411586589357392E-17, 0.000000000000000000, -1.000000000000000000 ) ) ;
#17286=CARTESIAN_POINT ( 'NONE',  ( -41.99999999999997868, 139.6861997365471950, 51.99999999999997868 ) ) ;
#17288=CARTESIAN_POINT ( 'NONE',  ( 46.99999999999998579, 115.0000000000000000, 37.49999999999997868 ) ) ;
#17291=VECTOR ( 'NONE', #247, 1000.000000000000000 ) ;
#17296=EDGE_CURVE ( 'NONE', #12653, #7321, #13629, .T. ) ;
#17303=DIRECTION ( 'NONE',  ( 1.000000000000000000, -0.000000000000000000, -0.000000000000000000 ) ) ;
#17320=CARTESIAN_POINT ( 'NONE',  ( -1.040834085586084257E-14, 27.62132034355962773, 54.62132034355965260 ) ) ;
#17322=DIRECTION ( 'NONE',  ( -0.000000000000000000, -1.000000000000000000, -0.000000000000000000 ) ) ;
#17342=ORIENTED_EDGE ( 'NONE', *, *, #17230, .F. ) ;
#17368=AXIS2_PLACEMENT_3D ( 'NONE', #9353, #12397, #8656 ) ;
#17392=EDGE_CURVE ( 'NONE', #4412, #12326, #16692, .T. ) ;
#17393=VECTOR ( 'NONE', #2079, 1000.000000000000000 ) ;
#17398=ORIENTED_EDGE ( 'NONE', *, *, #19206, .F. ) ;
#17399=EDGE_CURVE ( 'NONE', #6948, #15312, #18561, .T. ) ;
#17418=ADVANCED_FACE ( 'NONE', ( #9889 ), #17264, .F. ) ;
#17431=CARTESIAN_POINT ( 'NONE',  ( -1.040834085586084257E-14, 27.62132034355962773, 54.62132034355965260 ) ) ;
#17439=DIRECTION ( 'NONE',  ( -4.081702296416016490E-16, 0.000000000000000000, -1.000000000000000000 ) ) ;
#17441=ADVANCED_FACE ( 'NONE', ( #3732 ), #791, .F. ) ;
#17448=CARTESIAN_POINT ( 'NONE',  ( -2.750000000000023093, 118.0000000000000284, 37.49999999999997868 ) ) ;
#17493=EDGE_CURVE ( 'NONE', #8707, #4048, #15829, .T. ) ;
#17498=CIRCLE ( 'NONE', #6565, 1.500000000000001332 ) ;
#17502=FACE_OUTER_BOUND ( 'NONE', #18712, .T. ) ;
#17508=CARTESIAN_POINT ( 'NONE',  ( -1.040834085586084257E-14, 23.37867965644034030, 50.37867965644033319 ) ) ;
#17509=ORIENTED_EDGE ( 'NONE', *, *, #11511, .T. ) ;
#17535=CIRCLE ( 'NONE', #18787, 1.500000000000001332 ) ;
#17537=PLANE ( 'NONE',  #10020 ) ;
#17549=CARTESIAN_POINT ( 'NONE',  ( 2.749999999999981792, 118.0000000000000284, 37.49999999999997868 ) ) ;
#17551=EDGE_CURVE ( 'NONE', #19093, #17940, #7144, .T. ) ;
#17564=PRODUCT_CONTEXT ( 'NONE', #5081, 'mechanical' ) ;
#17580=AXIS2_PLACEMENT_3D ( 'NONE', #780, #3912, #8247 ) ;
#17581=CYLINDRICAL_SURFACE ( 'NONE', #6892, 6.000000000000000888 ) ;
#17585=CARTESIAN_POINT ( 'NONE',  ( -44.99999999999998579, 6.000000000000000000, -53.50000000000000000 ) ) ;
#17610=DIRECTION ( 'NONE',  ( 0.000000000000000000, 0.7071067811865492381, -0.7071067811865456854 ) ) ;
#17617=ORIENTED_EDGE ( 'NONE', *, *, #8210, .T. ) ;
#17630=DIRECTION ( 'NONE',  ( 0.000000000000000000, 0.000000000000000000, -1.000000000000000000 ) ) ;
#17636=CYLINDRICAL_SURFACE ( 'NONE', #178, 1.500000000000001332 ) ;
#17655=LINE ( 'NONE', #13133, #10656 ) ;
#17662=LINE ( 'NONE', #14721, #4245 ) ;
#17665=ADVANCED_FACE ( 'NONE', ( #94 ), #5875, .T. ) ;
#17715=VERTEX_POINT ( 'NONE', #14800 ) ;
#17739=EDGE_CURVE ( 'NONE', #12535, #18711, #4511, .T. ) ;
#17746=ADVANCED_FACE ( 'NONE', ( #5686 ), #17636, .F. ) ;
#17759=DIRECTION ( 'NONE',  ( -0.000000000000000000, 1.000000000000000000, 1.632680918566406547E-16 ) ) ;
#17810=VERTEX_POINT ( 'NONE', #14000 ) ;
#17866=CARTESIAN_POINT ( 'NONE',  ( -50.00000000000002132, 3.000000000000000000, -60.00000000000002132 ) ) ;
#17880=ORIENTED_EDGE ( 'NONE', *, *, #7464, .T. ) ;
#17915=LINE ( 'NONE', #11713, #813 ) ;
#17920=CARTESIAN_POINT ( 'NONE',  ( 2.749999999999979128, 118.0000000000000142, 40.49999999999995737 ) ) ;
#17924=DIRECTION ( 'NONE',  ( -0.000000000000000000, -1.000000000000000000, -0.000000000000000000 ) ) ;
#17933=EDGE_LOOP ( 'NONE', ( #8591, #8714, #13116, #14679 ) ) ;
#17940=VERTEX_POINT ( 'NONE', #11052 ) ;
#17946=ORIENTED_EDGE ( 'NONE', *, *, #11406, .T. ) ;
#17972=EDGE_LOOP ( 'NONE', ( #801, #16071, #18057, #16147 ) ) ;
#17973=CARTESIAN_POINT ( 'NONE',  ( -44.99999999999998579, 3.000000000000000000, -55.00000000000000000 ) ) ;
#18001=CARTESIAN_POINT ( 'NONE',  ( -1.040834085586084257E-14, 25.49999999999998934, 52.50000000000000711 ) ) ;
#18004=EDGE_CURVE ( 'NONE', #4631, #6552, #12534, .T. ) ;
#18006=VECTOR ( 'NONE', #10190, 1000.000000000000000 ) ;
#18017=ADVANCED_FACE ( 'NONE', ( #17236 ), #948, .T. ) ;
#18021=AXIS2_PLACEMENT_3D ( 'NONE', #13217, #16260, #11837 ) ;
#18023=DIRECTION ( 'NONE',  ( 0.000000000000000000, 0.7071067811865494601, -0.7071067811865456854 ) ) ;
#18028=DIRECTION ( 'NONE',  ( -1.000000000000000000, 0.000000000000000000, -6.672013369141567928E-17 ) ) ;
#18030=CARTESIAN_POINT ( 'NONE',  ( 41.99999999999997868, 6.000000000000005329, 51.99999999999997868 ) ) ;
#18031=CARTESIAN_POINT ( 'NONE',  ( 44.99999999999997158, 6.000000000000000000, 53.50000000000000000 ) ) ;
#18042=EDGE_CURVE ( 'NONE', #9683, #18948, #2141, .T. ) ;
#18047=ORIENTED_EDGE ( 'NONE', *, *, #3882, .T. ) ;
#18056=PLANE ( 'NONE',  #4071 ) ;
#18057=ORIENTED_EDGE ( 'NONE', *, *, #12764, .T. ) ;
#18096=CARTESIAN_POINT ( 'NONE',  ( -44.99999999999998579, 3.000000000000000000, -55.00000000000000000 ) ) ;
#18121=ORIENTED_EDGE ( 'NONE', *, *, #3159, .T. ) ;
#18144=EDGE_CURVE ( 'NONE', #2359, #5315, #17915, .T. ) ;
#18152=LINE ( 'NONE', #18256, #7 ) ;
#18178=DIRECTION ( 'NONE',  ( 1.000000000000000000, -0.000000000000000000, 0.000000000000000000 ) ) ;
#18207=LINE ( 'NONE', #19277, #18483 ) ;
#18213=EDGE_CURVE ( 'NONE', #14054, #6948, #8682, .T. ) ;
#18225=ORIENTED_EDGE ( 'NONE', *, *, #17551, .T. ) ;
#18230=VERTEX_POINT ( 'NONE', #16232 ) ;
#18238=VERTEX_POINT ( 'NONE', #16341 ) ;
#18250=FACE_OUTER_BOUND ( 'NONE', #7624, .T. ) ;
#18254=FILL_AREA_STYLE_COLOUR ( '', #2519 ) ;
#18256=CARTESIAN_POINT ( 'NONE',  ( 46.99999999999998579, 6.000000000000005329, 59.99999999999997868 ) ) ;
#18266=EDGE_CURVE ( 'NONE', #2159, #15084, #8953, .T. ) ;
#18283=CARTESIAN_POINT ( 'NONE',  ( -1.040834085586084257E-14, 27.62132034355962773, 54.62132034355965260 ) ) ;
#18286=CARTESIAN_POINT ( 'NONE',  ( -50.00000000000002132, 118.0000000000000142, 40.49999999999997868 ) ) ;
#18324=LINE ( 'NONE', #4894, #10350 ) ;
#18354=CYLINDRICAL_SURFACE ( 'NONE', #5800, 1.500000000000001332 ) ;
#18404=LINE ( 'NONE', #7807, #16013 ) ;
#18422=VERTEX_POINT ( 'NONE', #814 ) ;
#18442=ORIENTED_EDGE ( 'NONE', *, *, #18042, .F. ) ;
#18446=ORIENTED_EDGE ( 'NONE', *, *, #16711, .F. ) ;
#18462=VERTEX_POINT ( 'NONE', #17288 ) ;
#18465=CIRCLE ( 'NONE', #7800, 7.000000000000004441 ) ;
#18481=VECTOR ( 'NONE', #4844, 1000.000000000000000 ) ;
#18483=VECTOR ( 'NONE', #7507, 1000.000000000000000 ) ;
#18484=ORIENTED_EDGE ( 'NONE', *, *, #10674, .F. ) ;
#18495=VECTOR ( 'NONE', #1779, 1000.000000000000000 ) ;
#18499=CARTESIAN_POINT ( 'NONE',  ( -2.750000000000020872, 118.0000000000000142, 37.49999999999997158 ) ) ;
#18514=DIRECTION ( 'NONE',  ( 0.000000000000000000, -1.000000000000000000, 0.000000000000000000 ) ) ;
#18521=CARTESIAN_POINT ( 'NONE',  ( -50.00000000000002132, 118.0000000000000142, 37.49999999999997868 ) ) ;
#18528=DIRECTION ( 'NONE',  ( 5.782411586589357392E-17, -0.000000000000000000, 1.000000000000000000 ) ) ;
#18545=ORIENTED_EDGE ( 'NONE', *, *, #8362, .F. ) ;
#18553=CARTESIAN_POINT ( 'NONE',  ( -50.00000000000002132, 118.0000000000000142, 37.49999999999997868 ) ) ;
#18561=LINE ( 'NONE', #13736, #12389 ) ;
#18562=ORIENTED_EDGE ( 'NONE', *, *, #5773, .F. ) ;
#18571=LINE ( 'NONE', #11094, #2178 ) ;
#18601=FILL_AREA_STYLE ('',( #17034 ) ) ;
#18624=ORIENTED_EDGE ( 'NONE', *, *, #4091, .T. ) ;
#18635=CARTESIAN_POINT ( 'NONE',  ( -50.00000000000002132, 33.00000000000000000, 59.99999999999997868 ) ) ;
#18636=ORIENTED_EDGE ( 'NONE', *, *, #5881, .T. ) ;
#18639=DIRECTION ( 'NONE',  ( -4.088782444488986608E-17, 0.7071067811865495711, -0.7071067811865455743 ) ) ;
#18654=ORIENTED_EDGE ( 'NONE', *, *, #14543, .T. ) ;
#18659=DIRECTION ( 'NONE',  ( -3.826732013112564095E-16, 1.000000000000000000, 1.632680918566406793E-16 ) ) ;
#18673=CARTESIAN_POINT ( 'NONE',  ( 0.000000000000000000, 118.0000000000000142, 0.000000000000000000 ) ) ;
#18696=SURFACE_STYLE_FILL_AREA ( #18601 ) ;
#18711=VERTEX_POINT ( 'NONE', #3057 ) ;
#18712=EDGE_LOOP ( 'NONE', ( #14040, #2760 ) ) ;
#18716=VERTEX_POINT ( 'NONE', #10400 ) ;
#18741=DIRECTION ( 'NONE',  ( 0.000000000000000000, 0.7071067811865494601, -0.7071067811865455743 ) ) ;
#18743=ORIENTED_EDGE ( 'NONE', *, *, #4629, .T. ) ;
#18756=FACE_BOUND ( 'NONE', #196, .T. ) ;
#18787=AXIS2_PLACEMENT_3D ( 'NONE', #18819, #970, #11349 ) ;
#18797=CARTESIAN_POINT ( 'NONE',  ( -2.750000000000020872, 118.0000000000000142, 40.49999999999995737 ) ) ;
#18806=EDGE_LOOP ( 'NONE', ( #15360, #8552 ) ) ;
#18815=ORIENTED_EDGE ( 'NONE', *, *, #5328, .T. ) ;
#18819=CARTESIAN_POINT ( 'NONE',  ( -45.00000000000000000, 3.000000000000000000, 54.99999999999998579 ) ) ;
#18852=CARTESIAN_POINT ( 'NONE',  ( 44.99999999999998579, 3.000000000000000000, -56.49999999999998579 ) ) ;
#18862=ADVANCED_FACE ( 'NONE', ( #16994, #13939 ), #3454, .T. ) ;
#18875=EDGE_CURVE ( 'NONE', #10175, #12225, #709, .T. ) ;
#18879=CARTESIAN_POINT ( 'NONE',  ( 44.99999999999997158, 3.000000000000000000, 53.50000000000000000 ) ) ;
#18893=DIRECTION ( 'NONE',  ( 0.000000000000000000, -0.7071067811865492381, 0.7071067811865457964 ) ) ;
#18895=CARTESIAN_POINT ( 'NONE',  ( 44.99999999999998579, 3.000000000000000000, -54.99999999999998579 ) ) ;
#18901=ORIENTED_EDGE ( 'NONE', *, *, #888, .T. ) ;
#18911=ORIENTED_EDGE ( 'NONE', *, *, #19018, .T. ) ;
#18914=PLANE ( 'NONE',  #17580 ) ;
#18928=CARTESIAN_POINT ( 'NONE',  ( 46.99999999999998579, 30.00000000000000355, 37.49999999999996447 ) ) ;
#18937=LINE ( 'NONE', #11564, #9852 ) ;
#18944=FACE_OUTER_BOUND ( 'NONE', #9300, .T. ) ;
#18948=VERTEX_POINT ( 'NONE', #604 ) ;
#18994=EDGE_CURVE ( 'NONE', #6595, #5928, #5529, .T. ) ;
#19002=LINE ( 'NONE', #16054, #15719 ) ;
#19013=FACE_OUTER_BOUND ( 'NONE', #11068, .T. ) ;
#19018=EDGE_CURVE ( 'NONE', #869, #5315, #11456, .T. ) ;
#19021=ORIENTED_EDGE ( 'NONE', *, *, #148, .F. ) ;
#19023=CARTESIAN_POINT ( 'NONE',  ( -47.00000000000002132, 115.0000000000000000, -60.00000000000002132 ) ) ;
#19052=CARTESIAN_POINT ( 'NONE',  ( 2.750000000000009770, 38.00000000000000000, 40.49999999999995737 ) ) ;
#19080=EDGE_CURVE ( 'NONE', #6552, #15077, #14605, .T. ) ;
#19084=VECTOR ( 'NONE', #10178, 1000.000000000000000 ) ;
#19093=VERTEX_POINT ( 'NONE', #17175 ) ;
#19099=CYLINDRICAL_SURFACE ( 'NONE', #12813, 1.500000000000001332 ) ;
#19107=PLANE ( 'NONE',  #2487 ) ;
#19116=ORIENTED_EDGE ( 'NONE', *, *, #13456, .T. ) ;
#19119=DIRECTION ( 'NONE',  ( -0.000000000000000000, -1.000000000000000000, -0.000000000000000000 ) ) ;
#19140=LINE ( 'NONE', #17866, #2367 ) ;
#19176=CARTESIAN_POINT ( 'NONE',  ( 41.99999999999998579, 3.000000000000002665, -52.00000000000000000 ) ) ;
#19194=CYLINDRICAL_SURFACE ( 'NONE', #6018, 1.500000000000001332 ) ;
#19198=ADVANCED_FACE ( 'NONE', ( #14316 ), #884, .T. ) ;
#19206=EDGE_CURVE ( 'NONE', #2670, #4041, #16265, .T. ) ;
#19216=ORIENTED_EDGE ( 'NONE', *, *, #18042, .T. ) ;
#19277=CARTESIAN_POINT ( 'NONE',  ( 2.749999999999979128, 118.0000000000000000, 37.49999999999997158 ) ) ;
#19308=EDGE_CURVE ( 'NONE', #5915, #1741, #4936, .T. ) ;
#19346=ORIENTED_EDGE ( 'NONE', *, *, #665, .T. ) ;
#19348=ORIENTED_EDGE ( 'NONE', *, *, #8035, .T. ) ;
#19367=CARTESIAN_POINT ( 'NONE',  ( 43.50000000000001421, 115.0000000000000000, 32.49999999999998579 ) ) ;
#19371=CYLINDRICAL_SURFACE ( 'NONE', #607, 1.500000000000001332 ) ;
#19374=LINE ( 'NONE', #2704, #3182 ) ;
ENDSEC;
END-ISO-10303-21;
